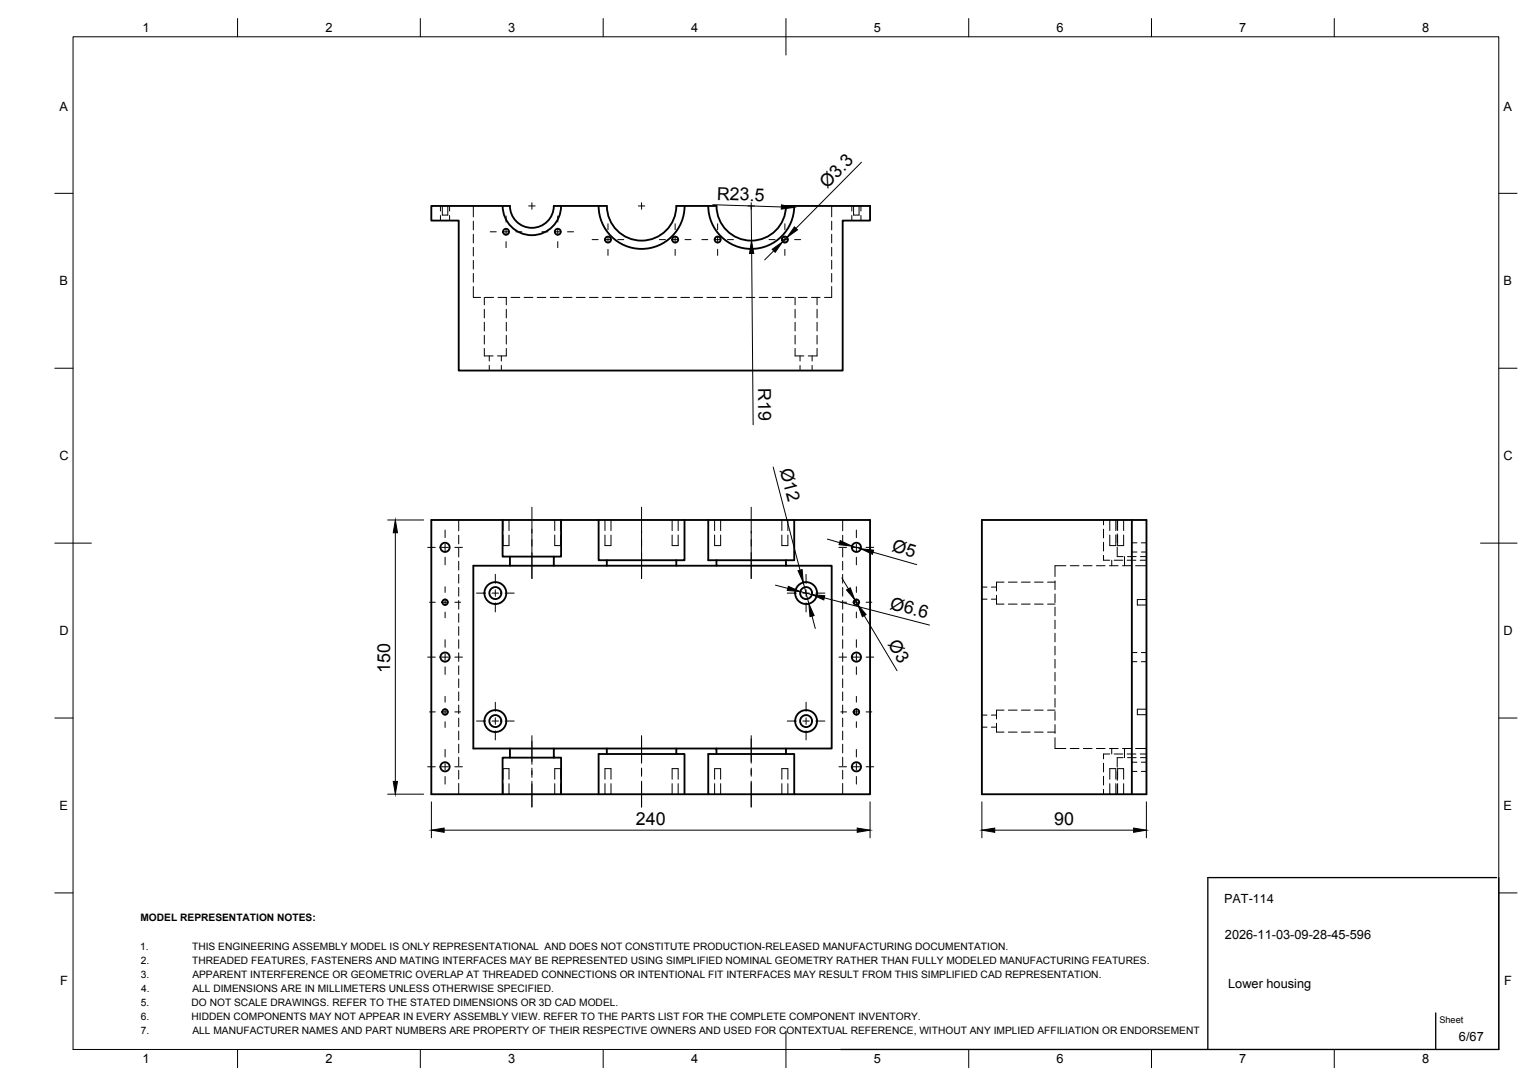
ISO-10303-21;
HEADER;
/* Generated by software containing ST-Developer
 * from STEP Tools, Inc. (www.steptools.com) 
 */

FILE_DESCRIPTION(
/* description */ ('Two-stage gear reducer in split housing'),
/* implementation_level */ '2;1');

FILE_NAME(
/* name */ 'Lower housing.step',
/* time_stamp */ '2026-10-28T03:22:31-07:00',
/* author */ (''),
/* organization */ (''),
/* preprocessor_version */ 'ST-DEVELOPER v20.2',
/* originating_system */ 'Autodesk Translation Framework v15.17.0.0',
/* authorisation */ '');

FILE_SCHEMA (('AUTOMOTIVE_DESIGN { 1 0 10303 214 3 1 1 }'));
ENDSEC;

DATA;
#10=MECHANICAL_DESIGN_GEOMETRIC_PRESENTATION_REPRESENTATION('',(#1235),#73366);
#1123=SHAPE_REPRESENTATION_RELATIONSHIP('SRR','None',#73610,#1179);
#1179=ADVANCED_BREP_SHAPE_REPRESENTATION('',(#1306),#73306);
#1235=STYLED_ITEM('',(#73967),#1306);
#1306=MANIFOLD_SOLID_BREP('Body1',#16123);
#1382=FACE_BOUND('',#2944,.T.);
#1383=FACE_BOUND('',#2945,.T.);
#1384=FACE_BOUND('',#2946,.T.);
#1385=FACE_BOUND('',#2947,.T.);
#1386=FACE_BOUND('',#2948,.T.);
#1387=FACE_BOUND('',#2949,.T.);
#1388=FACE_BOUND('',#2951,.T.);
#1389=FACE_BOUND('',#2952,.T.);
#1390=FACE_BOUND('',#2953,.T.);
#1391=FACE_BOUND('',#2954,.T.);
#1392=FACE_BOUND('',#2955,.T.);
#1393=FACE_BOUND('',#2959,.T.);
#1394=FACE_BOUND('',#2960,.T.);
#1395=FACE_BOUND('',#2961,.T.);
#1396=FACE_BOUND('',#2962,.T.);
#1397=FACE_BOUND('',#2963,.T.);
#1398=FACE_BOUND('',#2964,.T.);
#1399=FACE_BOUND('',#2998,.T.);
#1400=FACE_BOUND('',#2999,.T.);
#1401=FACE_BOUND('',#3000,.T.);
#1402=FACE_BOUND('',#3001,.T.);
#1403=FACE_BOUND('',#3002,.T.);
#1404=FACE_BOUND('',#3009,.T.);
#1405=FACE_BOUND('',#3012,.T.);
#1406=FACE_BOUND('',#3015,.T.);
#1407=FACE_BOUND('',#3018,.T.);
#1408=FACE_BOUND('',#3039,.T.);
#1409=FACE_BOUND('',#3040,.T.);
#1410=FACE_BOUND('',#3041,.T.);
#1411=FACE_BOUND('',#3045,.T.);
#1412=FACE_BOUND('',#3046,.T.);
#1413=FACE_BOUND('',#3047,.T.);
#1414=FACE_BOUND('',#3051,.T.);
#1415=FACE_BOUND('',#3052,.T.);
#1416=FACE_BOUND('',#3053,.T.);
#1417=FACE_BOUND('',#3054,.T.);
#1418=FACE_BOUND('',#3057,.T.);
#1419=FACE_BOUND('',#3058,.T.);
#1420=FACE_BOUND('',#3059,.T.);
#1421=FACE_BOUND('',#3060,.T.);
#1608=PLANE('',#16837);
#1609=PLANE('',#16841);
#1610=PLANE('',#16845);
#1611=PLANE('',#16849);
#1612=PLANE('',#16853);
#1613=PLANE('',#16855);
#1614=PLANE('',#16862);
#1615=PLANE('',#16871);
#1616=PLANE('',#16873);
#1617=PLANE('',#16880);
#1618=PLANE('',#16885);
#1619=PLANE('',#16888);
#1620=PLANE('',#16891);
#1621=PLANE('',#16894);
#1622=PLANE('',#16897);
#1623=PLANE('',#16900);
#1624=PLANE('',#16903);
#1625=PLANE('',#16907);
#1626=PLANE('',#16909);
#1627=PLANE('',#16913);
#1628=PLANE('',#16915);
#1629=PLANE('',#16918);
#1630=PLANE('',#16921);
#1631=PLANE('',#16924);
#1632=PLANE('',#16927);
#1633=PLANE('',#16930);
#1634=PLANE('',#16932);
#1635=PLANE('',#16940);
#1636=PLANE('',#16947);
#1637=PLANE('',#16952);
#1638=PLANE('',#16957);
#1639=PLANE('',#16962);
#1640=PLANE('',#16974);
#1641=PLANE('',#16977);
#1642=PLANE('',#16980);
#1643=PLANE('',#16983);
#1644=PLANE('',#16996);
#1645=PLANE('',#16997);
#1646=PLANE('',#16998);
#1647=PLANE('',#16999);
#1648=PLANE('',#17000);
#1649=PLANE('',#17001);
#1650=PLANE('',#17002);
#1651=PLANE('',#17003);
#1652=PLANE('',#17004);
#1653=PLANE('',#17005);
#2012=FACE_OUTER_BOUND('',#2933,.T.);
#2013=FACE_OUTER_BOUND('',#2934,.T.);
#2014=FACE_OUTER_BOUND('',#2935,.T.);
#2015=FACE_OUTER_BOUND('',#2936,.T.);
#2016=FACE_OUTER_BOUND('',#2937,.T.);
#2017=FACE_OUTER_BOUND('',#2938,.T.);
#2018=FACE_OUTER_BOUND('',#2939,.T.);
#2019=FACE_OUTER_BOUND('',#2940,.T.);
#2020=FACE_OUTER_BOUND('',#2941,.T.);
#2021=FACE_OUTER_BOUND('',#2942,.T.);
#2022=FACE_OUTER_BOUND('',#2943,.T.);
#2023=FACE_OUTER_BOUND('',#2950,.T.);
#2024=FACE_OUTER_BOUND('',#2956,.T.);
#2025=FACE_OUTER_BOUND('',#2957,.T.);
#2026=FACE_OUTER_BOUND('',#2958,.T.);
#2027=FACE_OUTER_BOUND('',#2965,.T.);
#2028=FACE_OUTER_BOUND('',#2966,.T.);
#2029=FACE_OUTER_BOUND('',#2967,.T.);
#2030=FACE_OUTER_BOUND('',#2968,.T.);
#2031=FACE_OUTER_BOUND('',#2969,.T.);
#2032=FACE_OUTER_BOUND('',#2970,.T.);
#2033=FACE_OUTER_BOUND('',#2971,.T.);
#2034=FACE_OUTER_BOUND('',#2972,.T.);
#2035=FACE_OUTER_BOUND('',#2973,.T.);
#2036=FACE_OUTER_BOUND('',#2974,.T.);
#2037=FACE_OUTER_BOUND('',#2975,.T.);
#2038=FACE_OUTER_BOUND('',#2976,.T.);
#2039=FACE_OUTER_BOUND('',#2977,.T.);
#2040=FACE_OUTER_BOUND('',#2978,.T.);
#2041=FACE_OUTER_BOUND('',#2979,.T.);
#2042=FACE_OUTER_BOUND('',#2980,.T.);
#2043=FACE_OUTER_BOUND('',#2981,.T.);
#2044=FACE_OUTER_BOUND('',#2982,.T.);
#2045=FACE_OUTER_BOUND('',#2983,.T.);
#2046=FACE_OUTER_BOUND('',#2984,.T.);
#2047=FACE_OUTER_BOUND('',#2985,.T.);
#2048=FACE_OUTER_BOUND('',#2986,.T.);
#2049=FACE_OUTER_BOUND('',#2987,.T.);
#2050=FACE_OUTER_BOUND('',#2988,.T.);
#2051=FACE_OUTER_BOUND('',#2989,.T.);
#2052=FACE_OUTER_BOUND('',#2990,.T.);
#2053=FACE_OUTER_BOUND('',#2991,.T.);
#2054=FACE_OUTER_BOUND('',#2992,.T.);
#2055=FACE_OUTER_BOUND('',#2993,.T.);
#2056=FACE_OUTER_BOUND('',#2994,.T.);
#2057=FACE_OUTER_BOUND('',#2995,.T.);
#2058=FACE_OUTER_BOUND('',#2996,.T.);
#2059=FACE_OUTER_BOUND('',#2997,.T.);
#2060=FACE_OUTER_BOUND('',#3003,.T.);
#2061=FACE_OUTER_BOUND('',#3004,.T.);
#2062=FACE_OUTER_BOUND('',#3005,.T.);
#2063=FACE_OUTER_BOUND('',#3006,.T.);
#2064=FACE_OUTER_BOUND('',#3007,.T.);
#2065=FACE_OUTER_BOUND('',#3008,.T.);
#2066=FACE_OUTER_BOUND('',#3010,.T.);
#2067=FACE_OUTER_BOUND('',#3011,.T.);
#2068=FACE_OUTER_BOUND('',#3013,.T.);
#2069=FACE_OUTER_BOUND('',#3014,.T.);
#2070=FACE_OUTER_BOUND('',#3016,.T.);
#2071=FACE_OUTER_BOUND('',#3017,.T.);
#2072=FACE_OUTER_BOUND('',#3019,.T.);
#2073=FACE_OUTER_BOUND('',#3020,.T.);
#2074=FACE_OUTER_BOUND('',#3021,.T.);
#2075=FACE_OUTER_BOUND('',#3022,.T.);
#2076=FACE_OUTER_BOUND('',#3023,.T.);
#2077=FACE_OUTER_BOUND('',#3024,.T.);
#2078=FACE_OUTER_BOUND('',#3025,.T.);
#2079=FACE_OUTER_BOUND('',#3026,.T.);
#2080=FACE_OUTER_BOUND('',#3027,.T.);
#2081=FACE_OUTER_BOUND('',#3028,.T.);
#2082=FACE_OUTER_BOUND('',#3029,.T.);
#2083=FACE_OUTER_BOUND('',#3030,.T.);
#2084=FACE_OUTER_BOUND('',#3031,.T.);
#2085=FACE_OUTER_BOUND('',#3032,.T.);
#2086=FACE_OUTER_BOUND('',#3033,.T.);
#2087=FACE_OUTER_BOUND('',#3034,.T.);
#2088=FACE_OUTER_BOUND('',#3035,.T.);
#2089=FACE_OUTER_BOUND('',#3036,.T.);
#2090=FACE_OUTER_BOUND('',#3037,.T.);
#2091=FACE_OUTER_BOUND('',#3038,.T.);
#2092=FACE_OUTER_BOUND('',#3042,.T.);
#2093=FACE_OUTER_BOUND('',#3043,.T.);
#2094=FACE_OUTER_BOUND('',#3044,.T.);
#2095=FACE_OUTER_BOUND('',#3048,.T.);
#2096=FACE_OUTER_BOUND('',#3049,.T.);
#2097=FACE_OUTER_BOUND('',#3050,.T.);
#2098=FACE_OUTER_BOUND('',#3055,.T.);
#2099=FACE_OUTER_BOUND('',#3056,.T.);
#2933=EDGE_LOOP('',(#10555,#10556,#10557,#10558));
#2934=EDGE_LOOP('',(#10559));
#2935=EDGE_LOOP('',(#10560,#10561,#10562,#10563));
#2936=EDGE_LOOP('',(#10564));
#2937=EDGE_LOOP('',(#10565,#10566,#10567,#10568));
#2938=EDGE_LOOP('',(#10569));
#2939=EDGE_LOOP('',(#10570,#10571,#10572,#10573));
#2940=EDGE_LOOP('',(#10574));
#2941=EDGE_LOOP('',(#10575,#10576,#10577,#10578));
#2942=EDGE_LOOP('',(#10579,#10580,#10581,#10582));
#2943=EDGE_LOOP('',(#10583,#10584,#10585,#10586,#10587,#10588,#10589,#10590,
#10591,#10592,#10593,#10594,#10595,#10596));
#2944=EDGE_LOOP('',(#10597));
#2945=EDGE_LOOP('',(#10598));
#2946=EDGE_LOOP('',(#10599));
#2947=EDGE_LOOP('',(#10600));
#2948=EDGE_LOOP('',(#10601));
#2949=EDGE_LOOP('',(#10602));
#2950=EDGE_LOOP('',(#10603,#10604,#10605,#10606,#10607,#10608,#10609,#10610,
#10611,#10612,#10613,#10614));
#2951=EDGE_LOOP('',(#10615));
#2952=EDGE_LOOP('',(#10616));
#2953=EDGE_LOOP('',(#10617));
#2954=EDGE_LOOP('',(#10618));
#2955=EDGE_LOOP('',(#10619));
#2956=EDGE_LOOP('',(#10620,#10621,#10622,#10623));
#2957=EDGE_LOOP('',(#10624,#10625,#10626,#10627));
#2958=EDGE_LOOP('',(#10628,#10629,#10630,#10631,#10632,#10633,#10634,#10635,
#10636,#10637,#10638,#10639,#10640,#10641));
#2959=EDGE_LOOP('',(#10642));
#2960=EDGE_LOOP('',(#10643));
#2961=EDGE_LOOP('',(#10644));
#2962=EDGE_LOOP('',(#10645));
#2963=EDGE_LOOP('',(#10646));
#2964=EDGE_LOOP('',(#10647));
#2965=EDGE_LOOP('',(#10648,#10649,#10650,#10651,#10652,#10653,#10654,#10655));
#2966=EDGE_LOOP('',(#10656,#10657,#10658,#10659));
#2967=EDGE_LOOP('',(#10660,#10661,#10662,#10663));
#2968=EDGE_LOOP('',(#10664,#10665,#10666,#10667,#10668,#10669,#10670,#10671,
#10672,#10673));
#2969=EDGE_LOOP('',(#10674,#10675,#10676,#10677,#10678,#10679,#10680,#10681));
#2970=EDGE_LOOP('',(#10682,#10683,#10684,#10685));
#2971=EDGE_LOOP('',(#10686));
#2972=EDGE_LOOP('',(#10687,#10688,#10689,#10690));
#2973=EDGE_LOOP('',(#10691));
#2974=EDGE_LOOP('',(#10692,#10693,#10694,#10695));
#2975=EDGE_LOOP('',(#10696));
#2976=EDGE_LOOP('',(#10697,#10698,#10699,#10700));
#2977=EDGE_LOOP('',(#10701));
#2978=EDGE_LOOP('',(#10702,#10703,#10704,#10705));
#2979=EDGE_LOOP('',(#10706,#10707,#10708,#10709));
#2980=EDGE_LOOP('',(#10710,#10711,#10712,#10713));
#2981=EDGE_LOOP('',(#10714,#10715,#10716,#10717));
#2982=EDGE_LOOP('',(#10718,#10719,#10720,#10721,#10722,#10723,#10724,#10725));
#2983=EDGE_LOOP('',(#10726,#10727,#10728,#10729));
#2984=EDGE_LOOP('',(#10730,#10731,#10732,#10733));
#2985=EDGE_LOOP('',(#10734,#10735,#10736,#10737,#10738,#10739,#10740,#10741,
#10742,#10743));
#2986=EDGE_LOOP('',(#10744,#10745,#10746,#10747,#10748,#10749,#10750,#10751));
#2987=EDGE_LOOP('',(#10752,#10753,#10754,#10755));
#2988=EDGE_LOOP('',(#10756));
#2989=EDGE_LOOP('',(#10757,#10758,#10759,#10760));
#2990=EDGE_LOOP('',(#10761));
#2991=EDGE_LOOP('',(#10762,#10763,#10764,#10765));
#2992=EDGE_LOOP('',(#10766));
#2993=EDGE_LOOP('',(#10767,#10768,#10769,#10770));
#2994=EDGE_LOOP('',(#10771));
#2995=EDGE_LOOP('',(#10772,#10773,#10774,#10775));
#2996=EDGE_LOOP('',(#10776,#10777,#10778,#10779));
#2997=EDGE_LOOP('',(#10780,#10781,#10782,#10783,#10784,#10785,#10786,#10787,
#10788,#10789,#10790,#10791));
#2998=EDGE_LOOP('',(#10792));
#2999=EDGE_LOOP('',(#10793));
#3000=EDGE_LOOP('',(#10794));
#3001=EDGE_LOOP('',(#10795));
#3002=EDGE_LOOP('',(#10796));
#3003=EDGE_LOOP('',(#10797,#10798,#10799,#10800));
#3004=EDGE_LOOP('',(#10801,#10802,#10803,#10804));
#3005=EDGE_LOOP('',(#10805,#10806,#10807,#10808));
#3006=EDGE_LOOP('',(#10809,#10810,#10811,#10812));
#3007=EDGE_LOOP('',(#10813,#10814,#10815,#10816));
#3008=EDGE_LOOP('',(#10817));
#3009=EDGE_LOOP('',(#10818));
#3010=EDGE_LOOP('',(#10819,#10820,#10821,#10822));
#3011=EDGE_LOOP('',(#10823));
#3012=EDGE_LOOP('',(#10824));
#3013=EDGE_LOOP('',(#10825,#10826,#10827,#10828));
#3014=EDGE_LOOP('',(#10829));
#3015=EDGE_LOOP('',(#10830));
#3016=EDGE_LOOP('',(#10831,#10832,#10833,#10834));
#3017=EDGE_LOOP('',(#10835));
#3018=EDGE_LOOP('',(#10836));
#3019=EDGE_LOOP('',(#10837,#10838,#10839,#10840));
#3020=EDGE_LOOP('',(#10841,#10842,#10843,#10844));
#3021=EDGE_LOOP('',(#10845,#10846,#10847,#10848));
#3022=EDGE_LOOP('',(#10849,#10850,#10851,#10852));
#3023=EDGE_LOOP('',(#10853,#10854,#10855,#10856));
#3024=EDGE_LOOP('',(#10857));
#3025=EDGE_LOOP('',(#10858,#10859,#10860,#10861));
#3026=EDGE_LOOP('',(#10862));
#3027=EDGE_LOOP('',(#10863,#10864,#10865,#10866));
#3028=EDGE_LOOP('',(#10867));
#3029=EDGE_LOOP('',(#10868,#10869,#10870,#10871));
#3030=EDGE_LOOP('',(#10872));
#3031=EDGE_LOOP('',(#10873,#10874,#10875,#10876));
#3032=EDGE_LOOP('',(#10877,#10878,#10879,#10880));
#3033=EDGE_LOOP('',(#10881,#10882,#10883,#10884));
#3034=EDGE_LOOP('',(#10885,#10886,#10887,#10888));
#3035=EDGE_LOOP('',(#10889,#10890,#10891,#10892));
#3036=EDGE_LOOP('',(#10893,#10894,#10895,#10896));
#3037=EDGE_LOOP('',(#10897,#10898,#10899,#10900));
#3038=EDGE_LOOP('',(#10901,#10902,#10903,#10904));
#3039=EDGE_LOOP('',(#10905));
#3040=EDGE_LOOP('',(#10906));
#3041=EDGE_LOOP('',(#10907));
#3042=EDGE_LOOP('',(#10908,#10909,#10910,#10911));
#3043=EDGE_LOOP('',(#10912,#10913,#10914,#10915));
#3044=EDGE_LOOP('',(#10916,#10917,#10918,#10919));
#3045=EDGE_LOOP('',(#10920));
#3046=EDGE_LOOP('',(#10921));
#3047=EDGE_LOOP('',(#10922));
#3048=EDGE_LOOP('',(#10923,#10924,#10925,#10926));
#3049=EDGE_LOOP('',(#10927,#10928,#10929,#10930));
#3050=EDGE_LOOP('',(#10931,#10932,#10933,#10934));
#3051=EDGE_LOOP('',(#10935));
#3052=EDGE_LOOP('',(#10936));
#3053=EDGE_LOOP('',(#10937));
#3054=EDGE_LOOP('',(#10938));
#3055=EDGE_LOOP('',(#10939,#10940,#10941,#10942));
#3056=EDGE_LOOP('',(#10943,#10944,#10945,#10946));
#3057=EDGE_LOOP('',(#10947));
#3058=EDGE_LOOP('',(#10948));
#3059=EDGE_LOOP('',(#10949));
#3060=EDGE_LOOP('',(#10950));
#4072=LINE('',#22832,#5096);
#4073=LINE('',#22839,#5097);
#4074=LINE('',#22846,#5098);
#4075=LINE('',#22853,#5099);
#4076=LINE('',#22859,#5100);
#4077=LINE('',#22863,#5101);
#4078=LINE('',#22867,#5102);
#4079=LINE('',#22870,#5103);
#4080=LINE('',#22873,#5104);
#4081=LINE('',#22875,#5105);
#4082=LINE('',#22877,#5106);
#4083=LINE('',#22879,#5107);
#4084=LINE('',#22881,#5108);
#4085=LINE('',#22883,#5109);
#4086=LINE('',#22885,#5110);
#4087=LINE('',#22887,#5111);
#4088=LINE('',#22889,#5112);
#4089=LINE('',#22893,#5113);
#4090=LINE('',#22896,#5114);
#4091=LINE('',#22907,#5115);
#4092=LINE('',#22909,#5116);
#4093=LINE('',#22911,#5117);
#4094=LINE('',#22913,#5118);
#4095=LINE('',#22915,#5119);
#4096=LINE('',#22917,#5120);
#4097=LINE('',#22919,#5121);
#4098=LINE('',#22921,#5122);
#4099=LINE('',#22922,#5123);
#4100=LINE('',#22937,#5124);
#4101=LINE('',#22942,#5125);
#4102=LINE('',#22945,#5126);
#4103=LINE('',#22949,#5127);
#4104=LINE('',#22953,#5128);
#4105=LINE('',#22955,#5129);
#4106=LINE('',#22957,#5130);
#4107=LINE('',#22959,#5131);
#4108=LINE('',#22961,#5132);
#4109=LINE('',#22963,#5133);
#4110=LINE('',#22965,#5134);
#4111=LINE('',#22966,#5135);
#4112=LINE('',#22977,#5136);
#4113=LINE('',#22979,#5137);
#4114=LINE('',#22981,#5138);
#4115=LINE('',#22983,#5139);
#4116=LINE('',#22984,#5140);
#4117=LINE('',#22989,#5141);
#4118=LINE('',#22993,#5142);
#4119=LINE('',#22997,#5143);
#4120=LINE('',#23001,#5144);
#4121=LINE('',#23003,#5145);
#4122=LINE('',#23005,#5146);
#4123=LINE('',#23006,#5147);
#4124=LINE('',#23009,#5148);
#4125=LINE('',#23011,#5149);
#4126=LINE('',#23012,#5150);
#4127=LINE('',#23016,#5151);
#4128=LINE('',#23021,#5152);
#4129=LINE('',#23025,#5153);
#4130=LINE('',#23030,#5154);
#4131=LINE('',#23035,#5155);
#4132=LINE('',#23039,#5156);
#4133=LINE('',#23044,#5157);
#4134=LINE('',#23048,#5158);
#4135=LINE('',#23051,#5159);
#4136=LINE('',#23053,#5160);
#4137=LINE('',#23055,#5161);
#4138=LINE('',#23057,#5162);
#4139=LINE('',#23058,#5163);
#4140=LINE('',#23060,#5164);
#4141=LINE('',#23065,#5165);
#4142=LINE('',#23067,#5166);
#4143=LINE('',#23069,#5167);
#4144=LINE('',#23071,#5168);
#4145=LINE('',#23075,#5169);
#4146=LINE('',#23077,#5170);
#4147=LINE('',#23078,#5171);
#4148=LINE('',#23082,#5172);
#4149=LINE('',#23087,#5173);
#4150=LINE('',#23091,#5174);
#4151=LINE('',#23096,#5175);
#4152=LINE('',#23101,#5176);
#4153=LINE('',#23105,#5177);
#4154=LINE('',#23108,#5178);
#4155=LINE('',#23110,#5179);
#4156=LINE('',#23112,#5180);
#4157=LINE('',#23113,#5181);
#4158=LINE('',#23114,#5182);
#4159=LINE('',#23115,#5183);
#4160=LINE('',#23136,#5184);
#4161=LINE('',#23145,#5185);
#4162=LINE('',#23154,#5186);
#4163=LINE('',#23163,#5187);
#4164=LINE('',#23171,#5188);
#4165=LINE('',#23175,#5189);
#4166=LINE('',#23179,#5190);
#4167=LINE('',#23183,#5191);
#4168=LINE('',#23187,#5192);
#4169=LINE('',#23192,#5193);
#4170=LINE('',#23197,#5194);
#4171=LINE('',#23202,#5195);
#4172=LINE('',#23207,#5196);
#4173=LINE('',#23211,#5197);
#4174=LINE('',#23215,#5198);
#4175=LINE('',#23219,#5199);
#4176=LINE('',#23223,#5200);
#4177=LINE('',#23227,#5201);
#4178=LINE('',#23229,#5202);
#4179=LINE('',#23231,#5203);
#4180=LINE('',#23233,#5204);
#4181=LINE('',#23235,#5205);
#4182=LINE('',#23237,#5206);
#4183=LINE('',#23239,#5207);
#4184=LINE('',#23241,#5208);
#4185=LINE('',#23244,#5209);
#5096=VECTOR('',#18522,0.164999999999999);
#5097=VECTOR('',#18531,0.164999999999999);
#5098=VECTOR('',#18540,0.164999999999999);
#5099=VECTOR('',#18549,0.164999999999999);
#5100=VECTOR('',#18556,1.);
#5101=VECTOR('',#18559,1.);
#5102=VECTOR('',#18564,1.);
#5103=VECTOR('',#18567,1.);
#5104=VECTOR('',#18570,1.);
#5105=VECTOR('',#18571,1.);
#5106=VECTOR('',#18572,1.);
#5107=VECTOR('',#18573,1.);
#5108=VECTOR('',#18574,1.);
#5109=VECTOR('',#18575,1.);
#5110=VECTOR('',#18576,1.);
#5111=VECTOR('',#18577,1.);
#5112=VECTOR('',#18578,1.);
#5113=VECTOR('',#18581,1.);
#5114=VECTOR('',#18584,1.);
#5115=VECTOR('',#18595,1.);
#5116=VECTOR('',#18596,1.);
#5117=VECTOR('',#18597,1.);
#5118=VECTOR('',#18598,1.);
#5119=VECTOR('',#18599,1.);
#5120=VECTOR('',#18600,1.);
#5121=VECTOR('',#18601,1.);
#5122=VECTOR('',#18602,1.);
#5123=VECTOR('',#18603,1.);
#5124=VECTOR('',#18618,1.);
#5125=VECTOR('',#18625,1.);
#5126=VECTOR('',#18628,1.);
#5127=VECTOR('',#18631,1.);
#5128=VECTOR('',#18634,1.);
#5129=VECTOR('',#18635,1.);
#5130=VECTOR('',#18636,1.);
#5131=VECTOR('',#18637,1.);
#5132=VECTOR('',#18638,1.);
#5133=VECTOR('',#18639,1.);
#5134=VECTOR('',#18640,1.);
#5135=VECTOR('',#18641,1.);
#5136=VECTOR('',#18652,1.);
#5137=VECTOR('',#18653,1.);
#5138=VECTOR('',#18654,1.);
#5139=VECTOR('',#18655,1.);
#5140=VECTOR('',#18656,1.);
#5141=VECTOR('',#18663,1.);
#5142=VECTOR('',#18668,1.);
#5143=VECTOR('',#18671,1.);
#5144=VECTOR('',#18674,1.);
#5145=VECTOR('',#18675,1.);
#5146=VECTOR('',#18676,1.);
#5147=VECTOR('',#18677,1.);
#5148=VECTOR('',#18680,1.);
#5149=VECTOR('',#18681,1.);
#5150=VECTOR('',#18682,1.);
#5151=VECTOR('',#18687,0.165);
#5152=VECTOR('',#18694,0.165);
#5153=VECTOR('',#18699,0.165);
#5154=VECTOR('',#18706,0.165);
#5155=VECTOR('',#18713,1.);
#5156=VECTOR('',#18718,1.);
#5157=VECTOR('',#18725,1.);
#5158=VECTOR('',#18730,1.);
#5159=VECTOR('',#18733,1.);
#5160=VECTOR('',#18734,1.);
#5161=VECTOR('',#18735,1.);
#5162=VECTOR('',#18736,1.);
#5163=VECTOR('',#18737,1.);
#5164=VECTOR('',#18740,1.);
#5165=VECTOR('',#18747,1.);
#5166=VECTOR('',#18748,1.);
#5167=VECTOR('',#18749,1.);
#5168=VECTOR('',#18750,1.);
#5169=VECTOR('',#18755,1.);
#5170=VECTOR('',#18756,1.);
#5171=VECTOR('',#18757,1.);
#5172=VECTOR('',#18762,0.165);
#5173=VECTOR('',#18769,0.165);
#5174=VECTOR('',#18774,0.165);
#5175=VECTOR('',#18781,0.165);
#5176=VECTOR('',#18788,1.);
#5177=VECTOR('',#18793,1.);
#5178=VECTOR('',#18798,1.);
#5179=VECTOR('',#18799,1.);
#5180=VECTOR('',#18800,1.);
#5181=VECTOR('',#18801,1.);
#5182=VECTOR('',#18802,1.);
#5183=VECTOR('',#18803,1.);
#5184=VECTOR('',#18830,0.6);
#5185=VECTOR('',#18841,0.6);
#5186=VECTOR('',#18852,0.6);
#5187=VECTOR('',#18863,0.6);
#5188=VECTOR('',#18874,0.33);
#5189=VECTOR('',#18879,0.33);
#5190=VECTOR('',#18884,0.33);
#5191=VECTOR('',#18889,0.33);
#5192=VECTOR('',#18894,0.149999999999999);
#5193=VECTOR('',#18901,0.149999999999999);
#5194=VECTOR('',#18908,0.15);
#5195=VECTOR('',#18915,0.15);
#5196=VECTOR('',#18922,0.25);
#5197=VECTOR('',#18927,0.25);
#5198=VECTOR('',#18932,0.25);
#5199=VECTOR('',#18937,0.25);
#5200=VECTOR('',#18942,0.25);
#5201=VECTOR('',#18947,0.25);
#5202=VECTOR('',#18950,1.);
#5203=VECTOR('',#18953,1.);
#5204=VECTOR('',#18956,1.);
#5205=VECTOR('',#18959,1.);
#5206=VECTOR('',#18962,1.);
#5207=VECTOR('',#18965,1.);
#5208=VECTOR('',#18968,1.);
#5209=VECTOR('',#18973,1.);
#6112=CIRCLE('',#16835,0.164999999999999);
#6113=CIRCLE('',#16836,0.164999999999999);
#6114=CIRCLE('',#16839,0.164999999999999);
#6115=CIRCLE('',#16840,0.164999999999999);
#6116=CIRCLE('',#16843,0.164999999999999);
#6117=CIRCLE('',#16844,0.164999999999999);
#6118=CIRCLE('',#16847,0.164999999999999);
#6119=CIRCLE('',#16848,0.164999999999999);
#6120=CIRCLE('',#16851,2.35);
#6121=CIRCLE('',#16852,2.35);
#6122=CIRCLE('',#16854,1.9);
#6123=CIRCLE('',#16856,1.6);
#6124=CIRCLE('',#16857,2.35);
#6125=CIRCLE('',#16858,0.165);
#6126=CIRCLE('',#16859,0.165);
#6127=CIRCLE('',#16860,0.165);
#6128=CIRCLE('',#16861,0.165);
#6129=CIRCLE('',#16863,0.149999999999999);
#6130=CIRCLE('',#16864,0.25);
#6131=CIRCLE('',#16865,0.25);
#6132=CIRCLE('',#16866,0.25);
#6133=CIRCLE('',#16867,0.149999999999999);
#6134=CIRCLE('',#16869,2.35);
#6135=CIRCLE('',#16870,2.35);
#6136=CIRCLE('',#16872,1.9);
#6137=CIRCLE('',#16874,2.35);
#6138=CIRCLE('',#16875,1.6);
#6139=CIRCLE('',#16876,0.165);
#6140=CIRCLE('',#16877,0.165);
#6141=CIRCLE('',#16878,0.165);
#6142=CIRCLE('',#16879,0.165);
#6143=CIRCLE('',#16882,1.9);
#6144=CIRCLE('',#16884,1.9);
#6145=CIRCLE('',#16886,1.9);
#6146=CIRCLE('',#16887,1.2);
#6147=CIRCLE('',#16890,0.165);
#6148=CIRCLE('',#16893,0.165);
#6149=CIRCLE('',#16896,0.165);
#6150=CIRCLE('',#16899,0.165);
#6151=CIRCLE('',#16902,2.35);
#6152=CIRCLE('',#16904,1.9);
#6153=CIRCLE('',#16906,2.35);
#6154=CIRCLE('',#16908,1.9);
#6155=CIRCLE('',#16912,1.9);
#6156=CIRCLE('',#16914,1.2);
#6157=CIRCLE('',#16917,0.165);
#6158=CIRCLE('',#16920,0.165);
#6159=CIRCLE('',#16923,0.165);
#6160=CIRCLE('',#16926,0.165);
#6161=CIRCLE('',#16929,1.6);
#6162=CIRCLE('',#16931,1.2);
#6163=CIRCLE('',#16933,0.15);
#6164=CIRCLE('',#16934,0.25);
#6165=CIRCLE('',#16935,0.25);
#6166=CIRCLE('',#16936,0.25);
#6167=CIRCLE('',#16937,0.15);
#6168=CIRCLE('',#16939,1.6);
#6169=CIRCLE('',#16941,1.2);
#6170=CIRCLE('',#16945,0.6);
#6171=CIRCLE('',#16946,0.6);
#6172=CIRCLE('',#16948,0.33);
#6173=CIRCLE('',#16950,0.6);
#6174=CIRCLE('',#16951,0.6);
#6175=CIRCLE('',#16953,0.33);
#6176=CIRCLE('',#16955,0.6);
#6177=CIRCLE('',#16956,0.6);
#6178=CIRCLE('',#16958,0.33);
#6179=CIRCLE('',#16960,0.6);
#6180=CIRCLE('',#16961,0.6);
#6181=CIRCLE('',#16963,0.33);
#6182=CIRCLE('',#16965,0.33);
#6183=CIRCLE('',#16967,0.33);
#6184=CIRCLE('',#16969,0.33);
#6185=CIRCLE('',#16971,0.33);
#6186=CIRCLE('',#16973,0.149999999999999);
#6187=CIRCLE('',#16976,0.149999999999999);
#6188=CIRCLE('',#16979,0.15);
#6189=CIRCLE('',#16982,0.15);
#6190=CIRCLE('',#16985,0.25);
#6191=CIRCLE('',#16987,0.25);
#6192=CIRCLE('',#16989,0.25);
#6193=CIRCLE('',#16991,0.25);
#6194=CIRCLE('',#16993,0.25);
#6195=CIRCLE('',#16995,0.25);
#6840=VERTEX_POINT('',#22829);
#6841=VERTEX_POINT('',#22831);
#6842=VERTEX_POINT('',#22836);
#6843=VERTEX_POINT('',#22838);
#6844=VERTEX_POINT('',#22843);
#6845=VERTEX_POINT('',#22845);
#6846=VERTEX_POINT('',#22850);
#6847=VERTEX_POINT('',#22852);
#6848=VERTEX_POINT('',#22857);
#6849=VERTEX_POINT('',#22858);
#6850=VERTEX_POINT('',#22860);
#6851=VERTEX_POINT('',#22862);
#6852=VERTEX_POINT('',#22866);
#6853=VERTEX_POINT('',#22868);
#6854=VERTEX_POINT('',#22872);
#6855=VERTEX_POINT('',#22874);
#6856=VERTEX_POINT('',#22876);
#6857=VERTEX_POINT('',#22878);
#6858=VERTEX_POINT('',#22880);
#6859=VERTEX_POINT('',#22882);
#6860=VERTEX_POINT('',#22884);
#6861=VERTEX_POINT('',#22886);
#6862=VERTEX_POINT('',#22888);
#6863=VERTEX_POINT('',#22890);
#6864=VERTEX_POINT('',#22892);
#6865=VERTEX_POINT('',#22894);
#6866=VERTEX_POINT('',#22897);
#6867=VERTEX_POINT('',#22899);
#6868=VERTEX_POINT('',#22901);
#6869=VERTEX_POINT('',#22903);
#6870=VERTEX_POINT('',#22906);
#6871=VERTEX_POINT('',#22908);
#6872=VERTEX_POINT('',#22910);
#6873=VERTEX_POINT('',#22912);
#6874=VERTEX_POINT('',#22914);
#6875=VERTEX_POINT('',#22916);
#6876=VERTEX_POINT('',#22918);
#6877=VERTEX_POINT('',#22920);
#6878=VERTEX_POINT('',#22923);
#6879=VERTEX_POINT('',#22925);
#6880=VERTEX_POINT('',#22927);
#6881=VERTEX_POINT('',#22929);
#6882=VERTEX_POINT('',#22931);
#6883=VERTEX_POINT('',#22934);
#6884=VERTEX_POINT('',#22936);
#6885=VERTEX_POINT('',#22940);
#6886=VERTEX_POINT('',#22944);
#6887=VERTEX_POINT('',#22946);
#6888=VERTEX_POINT('',#22948);
#6889=VERTEX_POINT('',#22950);
#6890=VERTEX_POINT('',#22952);
#6891=VERTEX_POINT('',#22954);
#6892=VERTEX_POINT('',#22956);
#6893=VERTEX_POINT('',#22958);
#6894=VERTEX_POINT('',#22960);
#6895=VERTEX_POINT('',#22962);
#6896=VERTEX_POINT('',#22964);
#6897=VERTEX_POINT('',#22967);
#6898=VERTEX_POINT('',#22969);
#6899=VERTEX_POINT('',#22971);
#6900=VERTEX_POINT('',#22973);
#6901=VERTEX_POINT('',#22976);
#6902=VERTEX_POINT('',#22978);
#6903=VERTEX_POINT('',#22980);
#6904=VERTEX_POINT('',#22982);
#6905=VERTEX_POINT('',#22988);
#6906=VERTEX_POINT('',#22992);
#6907=VERTEX_POINT('',#22994);
#6908=VERTEX_POINT('',#22996);
#6909=VERTEX_POINT('',#22998);
#6910=VERTEX_POINT('',#23000);
#6911=VERTEX_POINT('',#23002);
#6912=VERTEX_POINT('',#23004);
#6913=VERTEX_POINT('',#23008);
#6914=VERTEX_POINT('',#23010);
#6915=VERTEX_POINT('',#23014);
#6916=VERTEX_POINT('',#23019);
#6917=VERTEX_POINT('',#23024);
#6918=VERTEX_POINT('',#23029);
#6919=VERTEX_POINT('',#23034);
#6920=VERTEX_POINT('',#23038);
#6921=VERTEX_POINT('',#23042);
#6922=VERTEX_POINT('',#23046);
#6923=VERTEX_POINT('',#23050);
#6924=VERTEX_POINT('',#23052);
#6925=VERTEX_POINT('',#23054);
#6926=VERTEX_POINT('',#23056);
#6927=VERTEX_POINT('',#23064);
#6928=VERTEX_POINT('',#23066);
#6929=VERTEX_POINT('',#23068);
#6930=VERTEX_POINT('',#23070);
#6931=VERTEX_POINT('',#23074);
#6932=VERTEX_POINT('',#23076);
#6933=VERTEX_POINT('',#23080);
#6934=VERTEX_POINT('',#23085);
#6935=VERTEX_POINT('',#23090);
#6936=VERTEX_POINT('',#23095);
#6937=VERTEX_POINT('',#23100);
#6938=VERTEX_POINT('',#23104);
#6939=VERTEX_POINT('',#23109);
#6940=VERTEX_POINT('',#23111);
#6941=VERTEX_POINT('',#23116);
#6942=VERTEX_POINT('',#23118);
#6943=VERTEX_POINT('',#23120);
#6944=VERTEX_POINT('',#23122);
#6945=VERTEX_POINT('',#23124);
#6946=VERTEX_POINT('',#23133);
#6947=VERTEX_POINT('',#23135);
#6948=VERTEX_POINT('',#23139);
#6949=VERTEX_POINT('',#23142);
#6950=VERTEX_POINT('',#23144);
#6951=VERTEX_POINT('',#23148);
#6952=VERTEX_POINT('',#23151);
#6953=VERTEX_POINT('',#23153);
#6954=VERTEX_POINT('',#23157);
#6955=VERTEX_POINT('',#23160);
#6956=VERTEX_POINT('',#23162);
#6957=VERTEX_POINT('',#23166);
#6958=VERTEX_POINT('',#23169);
#6959=VERTEX_POINT('',#23173);
#6960=VERTEX_POINT('',#23177);
#6961=VERTEX_POINT('',#23181);
#6962=VERTEX_POINT('',#23185);
#6963=VERTEX_POINT('',#23190);
#6964=VERTEX_POINT('',#23195);
#6965=VERTEX_POINT('',#23200);
#6966=VERTEX_POINT('',#23205);
#6967=VERTEX_POINT('',#23209);
#6968=VERTEX_POINT('',#23213);
#6969=VERTEX_POINT('',#23217);
#6970=VERTEX_POINT('',#23221);
#6971=VERTEX_POINT('',#23225);
#8331=EDGE_CURVE('',#6840,#6840,#6112,.T.);
#8332=EDGE_CURVE('',#6840,#6841,#4072,.T.);
#8333=EDGE_CURVE('',#6841,#6841,#6113,.T.);
#8334=EDGE_CURVE('',#6842,#6842,#6114,.T.);
#8335=EDGE_CURVE('',#6842,#6843,#4073,.T.);
#8336=EDGE_CURVE('',#6843,#6843,#6115,.T.);
#8337=EDGE_CURVE('',#6844,#6844,#6116,.T.);
#8338=EDGE_CURVE('',#6844,#6845,#4074,.T.);
#8339=EDGE_CURVE('',#6845,#6845,#6117,.T.);
#8340=EDGE_CURVE('',#6846,#6846,#6118,.T.);
#8341=EDGE_CURVE('',#6846,#6847,#4075,.T.);
#8342=EDGE_CURVE('',#6847,#6847,#6119,.T.);
#8343=EDGE_CURVE('',#6848,#6849,#4076,.T.);
#8344=EDGE_CURVE('',#6850,#6848,#6120,.T.);
#8345=EDGE_CURVE('',#6851,#6850,#4077,.T.);
#8346=EDGE_CURVE('',#6849,#6851,#6121,.T.);
#8347=EDGE_CURVE('',#6852,#6848,#4078,.T.);
#8348=EDGE_CURVE('',#6853,#6852,#6122,.T.);
#8349=EDGE_CURVE('',#6850,#6853,#4079,.T.);
#8350=EDGE_CURVE('',#6854,#6851,#4080,.T.);
#8351=EDGE_CURVE('',#6855,#6854,#4081,.T.);
#8352=EDGE_CURVE('',#6855,#6856,#4082,.T.);
#8353=EDGE_CURVE('',#6857,#6856,#4083,.T.);
#8354=EDGE_CURVE('',#6857,#6858,#4084,.T.);
#8355=EDGE_CURVE('',#6858,#6859,#4085,.T.);
#8356=EDGE_CURVE('',#6859,#6860,#4086,.T.);
#8357=EDGE_CURVE('',#6860,#6861,#4087,.T.);
#8358=EDGE_CURVE('',#6862,#6861,#4088,.T.);
#8359=EDGE_CURVE('',#6862,#6863,#6123,.T.);
#8360=EDGE_CURVE('',#6864,#6863,#4089,.T.);
#8361=EDGE_CURVE('',#6864,#6865,#6124,.T.);
#8362=EDGE_CURVE('',#6849,#6865,#4090,.T.);
#8363=EDGE_CURVE('',#6866,#6866,#6125,.T.);
#8364=EDGE_CURVE('',#6867,#6867,#6126,.T.);
#8365=EDGE_CURVE('',#6868,#6868,#6127,.T.);
#8366=EDGE_CURVE('',#6869,#6869,#6128,.T.);
#8367=EDGE_CURVE('',#6853,#6870,#4091,.T.);
#8368=EDGE_CURVE('',#6870,#6871,#4092,.T.);
#8369=EDGE_CURVE('',#6871,#6872,#4093,.T.);
#8370=EDGE_CURVE('',#6872,#6873,#4094,.T.);
#8371=EDGE_CURVE('',#6873,#6874,#4095,.T.);
#8372=EDGE_CURVE('',#6874,#6875,#4096,.T.);
#8373=EDGE_CURVE('',#6875,#6876,#4097,.T.);
#8374=EDGE_CURVE('',#6876,#6877,#4098,.T.);
#8375=EDGE_CURVE('',#6877,#6854,#4099,.T.);
#8376=EDGE_CURVE('',#6878,#6878,#6129,.T.);
#8377=EDGE_CURVE('',#6879,#6879,#6130,.T.);
#8378=EDGE_CURVE('',#6880,#6880,#6131,.T.);
#8379=EDGE_CURVE('',#6881,#6881,#6132,.T.);
#8380=EDGE_CURVE('',#6882,#6882,#6133,.T.);
#8381=EDGE_CURVE('',#6875,#6883,#6134,.T.);
#8382=EDGE_CURVE('',#6884,#6883,#4100,.T.);
#8383=EDGE_CURVE('',#6876,#6884,#6135,.T.);
#8384=EDGE_CURVE('',#6885,#6874,#6136,.T.);
#8385=EDGE_CURVE('',#6883,#6885,#4101,.T.);
#8386=EDGE_CURVE('',#6886,#6884,#4102,.T.);
#8387=EDGE_CURVE('',#6886,#6887,#6137,.T.);
#8388=EDGE_CURVE('',#6888,#6887,#4103,.T.);
#8389=EDGE_CURVE('',#6888,#6889,#6138,.T.);
#8390=EDGE_CURVE('',#6890,#6889,#4104,.T.);
#8391=EDGE_CURVE('',#6891,#6890,#4105,.T.);
#8392=EDGE_CURVE('',#6891,#6892,#4106,.T.);
#8393=EDGE_CURVE('',#6893,#6892,#4107,.T.);
#8394=EDGE_CURVE('',#6893,#6894,#4108,.T.);
#8395=EDGE_CURVE('',#6894,#6895,#4109,.T.);
#8396=EDGE_CURVE('',#6895,#6896,#4110,.T.);
#8397=EDGE_CURVE('',#6896,#6877,#4111,.T.);
#8398=EDGE_CURVE('',#6897,#6897,#6139,.T.);
#8399=EDGE_CURVE('',#6898,#6898,#6140,.T.);
#8400=EDGE_CURVE('',#6899,#6899,#6141,.T.);
#8401=EDGE_CURVE('',#6900,#6900,#6142,.T.);
#8402=EDGE_CURVE('',#6885,#6901,#4112,.T.);
#8403=EDGE_CURVE('',#6901,#6902,#4113,.T.);
#8404=EDGE_CURVE('',#6902,#6903,#4114,.T.);
#8405=EDGE_CURVE('',#6903,#6904,#4115,.T.);
#8406=EDGE_CURVE('',#6904,#6886,#4116,.T.);
#8407=EDGE_CURVE('',#6901,#6873,#6143,.T.);
#8408=EDGE_CURVE('',#6905,#6852,#4117,.T.);
#8409=EDGE_CURVE('',#6870,#6905,#6144,.T.);
#8410=EDGE_CURVE('',#6906,#6905,#4118,.T.);
#8411=EDGE_CURVE('',#6906,#6907,#6145,.T.);
#8412=EDGE_CURVE('',#6908,#6907,#4119,.T.);
#8413=EDGE_CURVE('',#6908,#6909,#6146,.T.);
#8414=EDGE_CURVE('',#6910,#6909,#4120,.T.);
#8415=EDGE_CURVE('',#6911,#6910,#4121,.T.);
#8416=EDGE_CURVE('',#6912,#6911,#4122,.T.);
#8417=EDGE_CURVE('',#6912,#6871,#4123,.T.);
#8418=EDGE_CURVE('',#6865,#6913,#4124,.T.);
#8419=EDGE_CURVE('',#6913,#6914,#4125,.T.);
#8420=EDGE_CURVE('',#6914,#6906,#4126,.T.);
#8421=EDGE_CURVE('',#6915,#6915,#6147,.T.);
#8422=EDGE_CURVE('',#6915,#6869,#4127,.T.);
#8423=EDGE_CURVE('',#6916,#6916,#6148,.T.);
#8424=EDGE_CURVE('',#6916,#6868,#4128,.T.);
#8425=EDGE_CURVE('',#6897,#6917,#4129,.T.);
#8426=EDGE_CURVE('',#6917,#6917,#6149,.T.);
#8427=EDGE_CURVE('',#6898,#6918,#4130,.T.);
#8428=EDGE_CURVE('',#6918,#6918,#6150,.T.);
#8429=EDGE_CURVE('',#6919,#6864,#4131,.T.);
#8430=EDGE_CURVE('',#6913,#6919,#6151,.T.);
#8431=EDGE_CURVE('',#6920,#6919,#4132,.T.);
#8432=EDGE_CURVE('',#6914,#6920,#6152,.T.);
#8433=EDGE_CURVE('',#6904,#6921,#6153,.T.);
#8434=EDGE_CURVE('',#6887,#6921,#4133,.T.);
#8435=EDGE_CURVE('',#6922,#6903,#6154,.T.);
#8436=EDGE_CURVE('',#6921,#6922,#4134,.T.);
#8437=EDGE_CURVE('',#6922,#6923,#4135,.T.);
#8438=EDGE_CURVE('',#6923,#6924,#4136,.T.);
#8439=EDGE_CURVE('',#6924,#6925,#4137,.T.);
#8440=EDGE_CURVE('',#6925,#6926,#4138,.T.);
#8441=EDGE_CURVE('',#6926,#6888,#4139,.T.);
#8442=EDGE_CURVE('',#6907,#6920,#4140,.T.);
#8443=EDGE_CURVE('',#6923,#6902,#6155,.T.);
#8444=EDGE_CURVE('',#6927,#6872,#4141,.T.);
#8445=EDGE_CURVE('',#6928,#6927,#4142,.T.);
#8446=EDGE_CURVE('',#6928,#6929,#4143,.T.);
#8447=EDGE_CURVE('',#6930,#6929,#4144,.T.);
#8448=EDGE_CURVE('',#6930,#6924,#6156,.T.);
#8449=EDGE_CURVE('',#6863,#6931,#4145,.T.);
#8450=EDGE_CURVE('',#6931,#6932,#4146,.T.);
#8451=EDGE_CURVE('',#6932,#6908,#4147,.T.);
#8452=EDGE_CURVE('',#6933,#6933,#6157,.T.);
#8453=EDGE_CURVE('',#6933,#6867,#4148,.T.);
#8454=EDGE_CURVE('',#6934,#6934,#6158,.T.);
#8455=EDGE_CURVE('',#6934,#6866,#4149,.T.);
#8456=EDGE_CURVE('',#6900,#6935,#4150,.T.);
#8457=EDGE_CURVE('',#6935,#6935,#6159,.T.);
#8458=EDGE_CURVE('',#6899,#6936,#4151,.T.);
#8459=EDGE_CURVE('',#6936,#6936,#6160,.T.);
#8460=EDGE_CURVE('',#6937,#6862,#4152,.T.);
#8461=EDGE_CURVE('',#6931,#6937,#6161,.T.);
#8462=EDGE_CURVE('',#6938,#6937,#4153,.T.);
#8463=EDGE_CURVE('',#6932,#6938,#6162,.T.);
#8464=EDGE_CURVE('',#6861,#6890,#4154,.T.);
#8465=EDGE_CURVE('',#6889,#6939,#4155,.T.);
#8466=EDGE_CURVE('',#6939,#6940,#4156,.T.);
#8467=EDGE_CURVE('',#6940,#6930,#4157,.T.);
#8468=EDGE_CURVE('',#6929,#6910,#4158,.T.);
#8469=EDGE_CURVE('',#6909,#6938,#4159,.T.);
#8470=EDGE_CURVE('',#6941,#6941,#6163,.T.);
#8471=EDGE_CURVE('',#6942,#6942,#6164,.T.);
#8472=EDGE_CURVE('',#6943,#6943,#6165,.T.);
#8473=EDGE_CURVE('',#6944,#6944,#6166,.T.);
#8474=EDGE_CURVE('',#6945,#6945,#6167,.T.);
#8475=EDGE_CURVE('',#6926,#6939,#6168,.T.);
#8476=EDGE_CURVE('',#6940,#6925,#6169,.T.);
#8477=EDGE_CURVE('',#6946,#6946,#6170,.T.);
#8478=EDGE_CURVE('',#6946,#6947,#4160,.T.);
#8479=EDGE_CURVE('',#6947,#6947,#6171,.T.);
#8480=EDGE_CURVE('',#6948,#6948,#6172,.T.);
#8481=EDGE_CURVE('',#6949,#6949,#6173,.T.);
#8482=EDGE_CURVE('',#6949,#6950,#4161,.T.);
#8483=EDGE_CURVE('',#6950,#6950,#6174,.T.);
#8484=EDGE_CURVE('',#6951,#6951,#6175,.T.);
#8485=EDGE_CURVE('',#6952,#6952,#6176,.T.);
#8486=EDGE_CURVE('',#6952,#6953,#4162,.T.);
#8487=EDGE_CURVE('',#6953,#6953,#6177,.T.);
#8488=EDGE_CURVE('',#6954,#6954,#6178,.T.);
#8489=EDGE_CURVE('',#6955,#6955,#6179,.T.);
#8490=EDGE_CURVE('',#6955,#6956,#4163,.T.);
#8491=EDGE_CURVE('',#6956,#6956,#6180,.T.);
#8492=EDGE_CURVE('',#6957,#6957,#6181,.T.);
#8493=EDGE_CURVE('',#6958,#6958,#6182,.T.);
#8494=EDGE_CURVE('',#6958,#6948,#4164,.T.);
#8495=EDGE_CURVE('',#6959,#6959,#6183,.T.);
#8496=EDGE_CURVE('',#6959,#6951,#4165,.T.);
#8497=EDGE_CURVE('',#6960,#6960,#6184,.T.);
#8498=EDGE_CURVE('',#6960,#6954,#4166,.T.);
#8499=EDGE_CURVE('',#6961,#6961,#6185,.T.);
#8500=EDGE_CURVE('',#6961,#6957,#4167,.T.);
#8501=EDGE_CURVE('',#6962,#6962,#6186,.T.);
#8502=EDGE_CURVE('',#6962,#6878,#4168,.T.);
#8503=EDGE_CURVE('',#6963,#6963,#6187,.T.);
#8504=EDGE_CURVE('',#6963,#6882,#4169,.T.);
#8505=EDGE_CURVE('',#6964,#6964,#6188,.T.);
#8506=EDGE_CURVE('',#6964,#6941,#4170,.T.);
#8507=EDGE_CURVE('',#6965,#6965,#6189,.T.);
#8508=EDGE_CURVE('',#6965,#6945,#4171,.T.);
#8509=EDGE_CURVE('',#6966,#6966,#6190,.T.);
#8510=EDGE_CURVE('',#6966,#6879,#4172,.T.);
#8511=EDGE_CURVE('',#6967,#6967,#6191,.T.);
#8512=EDGE_CURVE('',#6967,#6942,#4173,.T.);
#8513=EDGE_CURVE('',#6968,#6968,#6192,.T.);
#8514=EDGE_CURVE('',#6968,#6943,#4174,.T.);
#8515=EDGE_CURVE('',#6969,#6969,#6193,.T.);
#8516=EDGE_CURVE('',#6969,#6944,#4175,.T.);
#8517=EDGE_CURVE('',#6970,#6970,#6194,.T.);
#8518=EDGE_CURVE('',#6970,#6880,#4176,.T.);
#8519=EDGE_CURVE('',#6971,#6971,#6195,.T.);
#8520=EDGE_CURVE('',#6971,#6881,#4177,.T.);
#8521=EDGE_CURVE('',#6896,#6855,#4178,.T.);
#8522=EDGE_CURVE('',#6856,#6895,#4179,.T.);
#8523=EDGE_CURVE('',#6894,#6857,#4180,.T.);
#8524=EDGE_CURVE('',#6860,#6891,#4181,.T.);
#8525=EDGE_CURVE('',#6892,#6859,#4182,.T.);
#8526=EDGE_CURVE('',#6911,#6928,#4183,.T.);
#8527=EDGE_CURVE('',#6927,#6912,#4184,.T.);
#8528=EDGE_CURVE('',#6858,#6893,#4185,.T.);
#10555=ORIENTED_EDGE('',*,*,#8331,.F.);
#10556=ORIENTED_EDGE('',*,*,#8332,.T.);
#10557=ORIENTED_EDGE('',*,*,#8333,.F.);
#10558=ORIENTED_EDGE('',*,*,#8332,.F.);
#10559=ORIENTED_EDGE('',*,*,#8331,.T.);
#10560=ORIENTED_EDGE('',*,*,#8334,.F.);
#10561=ORIENTED_EDGE('',*,*,#8335,.T.);
#10562=ORIENTED_EDGE('',*,*,#8336,.F.);
#10563=ORIENTED_EDGE('',*,*,#8335,.F.);
#10564=ORIENTED_EDGE('',*,*,#8334,.T.);
#10565=ORIENTED_EDGE('',*,*,#8337,.F.);
#10566=ORIENTED_EDGE('',*,*,#8338,.T.);
#10567=ORIENTED_EDGE('',*,*,#8339,.T.);
#10568=ORIENTED_EDGE('',*,*,#8338,.F.);
#10569=ORIENTED_EDGE('',*,*,#8339,.F.);
#10570=ORIENTED_EDGE('',*,*,#8340,.F.);
#10571=ORIENTED_EDGE('',*,*,#8341,.T.);
#10572=ORIENTED_EDGE('',*,*,#8342,.T.);
#10573=ORIENTED_EDGE('',*,*,#8341,.F.);
#10574=ORIENTED_EDGE('',*,*,#8342,.F.);
#10575=ORIENTED_EDGE('',*,*,#8343,.F.);
#10576=ORIENTED_EDGE('',*,*,#8344,.F.);
#10577=ORIENTED_EDGE('',*,*,#8345,.F.);
#10578=ORIENTED_EDGE('',*,*,#8346,.F.);
#10579=ORIENTED_EDGE('',*,*,#8347,.F.);
#10580=ORIENTED_EDGE('',*,*,#8348,.F.);
#10581=ORIENTED_EDGE('',*,*,#8349,.F.);
#10582=ORIENTED_EDGE('',*,*,#8344,.T.);
#10583=ORIENTED_EDGE('',*,*,#8346,.T.);
#10584=ORIENTED_EDGE('',*,*,#8350,.F.);
#10585=ORIENTED_EDGE('',*,*,#8351,.F.);
#10586=ORIENTED_EDGE('',*,*,#8352,.T.);
#10587=ORIENTED_EDGE('',*,*,#8353,.F.);
#10588=ORIENTED_EDGE('',*,*,#8354,.T.);
#10589=ORIENTED_EDGE('',*,*,#8355,.T.);
#10590=ORIENTED_EDGE('',*,*,#8356,.T.);
#10591=ORIENTED_EDGE('',*,*,#8357,.T.);
#10592=ORIENTED_EDGE('',*,*,#8358,.F.);
#10593=ORIENTED_EDGE('',*,*,#8359,.T.);
#10594=ORIENTED_EDGE('',*,*,#8360,.F.);
#10595=ORIENTED_EDGE('',*,*,#8361,.T.);
#10596=ORIENTED_EDGE('',*,*,#8362,.F.);
#10597=ORIENTED_EDGE('',*,*,#8333,.T.);
#10598=ORIENTED_EDGE('',*,*,#8336,.T.);
#10599=ORIENTED_EDGE('',*,*,#8363,.T.);
#10600=ORIENTED_EDGE('',*,*,#8364,.T.);
#10601=ORIENTED_EDGE('',*,*,#8365,.T.);
#10602=ORIENTED_EDGE('',*,*,#8366,.T.);
#10603=ORIENTED_EDGE('',*,*,#8345,.T.);
#10604=ORIENTED_EDGE('',*,*,#8349,.T.);
#10605=ORIENTED_EDGE('',*,*,#8367,.T.);
#10606=ORIENTED_EDGE('',*,*,#8368,.T.);
#10607=ORIENTED_EDGE('',*,*,#8369,.T.);
#10608=ORIENTED_EDGE('',*,*,#8370,.T.);
#10609=ORIENTED_EDGE('',*,*,#8371,.T.);
#10610=ORIENTED_EDGE('',*,*,#8372,.T.);
#10611=ORIENTED_EDGE('',*,*,#8373,.T.);
#10612=ORIENTED_EDGE('',*,*,#8374,.T.);
#10613=ORIENTED_EDGE('',*,*,#8375,.T.);
#10614=ORIENTED_EDGE('',*,*,#8350,.T.);
#10615=ORIENTED_EDGE('',*,*,#8376,.T.);
#10616=ORIENTED_EDGE('',*,*,#8377,.T.);
#10617=ORIENTED_EDGE('',*,*,#8378,.T.);
#10618=ORIENTED_EDGE('',*,*,#8379,.T.);
#10619=ORIENTED_EDGE('',*,*,#8380,.T.);
#10620=ORIENTED_EDGE('',*,*,#8373,.F.);
#10621=ORIENTED_EDGE('',*,*,#8381,.T.);
#10622=ORIENTED_EDGE('',*,*,#8382,.F.);
#10623=ORIENTED_EDGE('',*,*,#8383,.F.);
#10624=ORIENTED_EDGE('',*,*,#8372,.F.);
#10625=ORIENTED_EDGE('',*,*,#8384,.F.);
#10626=ORIENTED_EDGE('',*,*,#8385,.F.);
#10627=ORIENTED_EDGE('',*,*,#8381,.F.);
#10628=ORIENTED_EDGE('',*,*,#8383,.T.);
#10629=ORIENTED_EDGE('',*,*,#8386,.F.);
#10630=ORIENTED_EDGE('',*,*,#8387,.T.);
#10631=ORIENTED_EDGE('',*,*,#8388,.F.);
#10632=ORIENTED_EDGE('',*,*,#8389,.T.);
#10633=ORIENTED_EDGE('',*,*,#8390,.F.);
#10634=ORIENTED_EDGE('',*,*,#8391,.F.);
#10635=ORIENTED_EDGE('',*,*,#8392,.T.);
#10636=ORIENTED_EDGE('',*,*,#8393,.F.);
#10637=ORIENTED_EDGE('',*,*,#8394,.T.);
#10638=ORIENTED_EDGE('',*,*,#8395,.T.);
#10639=ORIENTED_EDGE('',*,*,#8396,.T.);
#10640=ORIENTED_EDGE('',*,*,#8397,.T.);
#10641=ORIENTED_EDGE('',*,*,#8374,.F.);
#10642=ORIENTED_EDGE('',*,*,#8337,.T.);
#10643=ORIENTED_EDGE('',*,*,#8340,.T.);
#10644=ORIENTED_EDGE('',*,*,#8398,.T.);
#10645=ORIENTED_EDGE('',*,*,#8399,.T.);
#10646=ORIENTED_EDGE('',*,*,#8400,.T.);
#10647=ORIENTED_EDGE('',*,*,#8401,.T.);
#10648=ORIENTED_EDGE('',*,*,#8382,.T.);
#10649=ORIENTED_EDGE('',*,*,#8385,.T.);
#10650=ORIENTED_EDGE('',*,*,#8402,.T.);
#10651=ORIENTED_EDGE('',*,*,#8403,.T.);
#10652=ORIENTED_EDGE('',*,*,#8404,.T.);
#10653=ORIENTED_EDGE('',*,*,#8405,.T.);
#10654=ORIENTED_EDGE('',*,*,#8406,.T.);
#10655=ORIENTED_EDGE('',*,*,#8386,.T.);
#10656=ORIENTED_EDGE('',*,*,#8384,.T.);
#10657=ORIENTED_EDGE('',*,*,#8371,.F.);
#10658=ORIENTED_EDGE('',*,*,#8407,.F.);
#10659=ORIENTED_EDGE('',*,*,#8402,.F.);
#10660=ORIENTED_EDGE('',*,*,#8348,.T.);
#10661=ORIENTED_EDGE('',*,*,#8408,.F.);
#10662=ORIENTED_EDGE('',*,*,#8409,.F.);
#10663=ORIENTED_EDGE('',*,*,#8367,.F.);
#10664=ORIENTED_EDGE('',*,*,#8409,.T.);
#10665=ORIENTED_EDGE('',*,*,#8410,.F.);
#10666=ORIENTED_EDGE('',*,*,#8411,.T.);
#10667=ORIENTED_EDGE('',*,*,#8412,.F.);
#10668=ORIENTED_EDGE('',*,*,#8413,.T.);
#10669=ORIENTED_EDGE('',*,*,#8414,.F.);
#10670=ORIENTED_EDGE('',*,*,#8415,.F.);
#10671=ORIENTED_EDGE('',*,*,#8416,.F.);
#10672=ORIENTED_EDGE('',*,*,#8417,.T.);
#10673=ORIENTED_EDGE('',*,*,#8368,.F.);
#10674=ORIENTED_EDGE('',*,*,#8343,.T.);
#10675=ORIENTED_EDGE('',*,*,#8362,.T.);
#10676=ORIENTED_EDGE('',*,*,#8418,.T.);
#10677=ORIENTED_EDGE('',*,*,#8419,.T.);
#10678=ORIENTED_EDGE('',*,*,#8420,.T.);
#10679=ORIENTED_EDGE('',*,*,#8410,.T.);
#10680=ORIENTED_EDGE('',*,*,#8408,.T.);
#10681=ORIENTED_EDGE('',*,*,#8347,.T.);
#10682=ORIENTED_EDGE('',*,*,#8421,.F.);
#10683=ORIENTED_EDGE('',*,*,#8422,.T.);
#10684=ORIENTED_EDGE('',*,*,#8366,.F.);
#10685=ORIENTED_EDGE('',*,*,#8422,.F.);
#10686=ORIENTED_EDGE('',*,*,#8421,.T.);
#10687=ORIENTED_EDGE('',*,*,#8423,.F.);
#10688=ORIENTED_EDGE('',*,*,#8424,.T.);
#10689=ORIENTED_EDGE('',*,*,#8365,.F.);
#10690=ORIENTED_EDGE('',*,*,#8424,.F.);
#10691=ORIENTED_EDGE('',*,*,#8423,.T.);
#10692=ORIENTED_EDGE('',*,*,#8398,.F.);
#10693=ORIENTED_EDGE('',*,*,#8425,.T.);
#10694=ORIENTED_EDGE('',*,*,#8426,.T.);
#10695=ORIENTED_EDGE('',*,*,#8425,.F.);
#10696=ORIENTED_EDGE('',*,*,#8426,.F.);
#10697=ORIENTED_EDGE('',*,*,#8399,.F.);
#10698=ORIENTED_EDGE('',*,*,#8427,.T.);
#10699=ORIENTED_EDGE('',*,*,#8428,.T.);
#10700=ORIENTED_EDGE('',*,*,#8427,.F.);
#10701=ORIENTED_EDGE('',*,*,#8428,.F.);
#10702=ORIENTED_EDGE('',*,*,#8429,.F.);
#10703=ORIENTED_EDGE('',*,*,#8430,.F.);
#10704=ORIENTED_EDGE('',*,*,#8418,.F.);
#10705=ORIENTED_EDGE('',*,*,#8361,.F.);
#10706=ORIENTED_EDGE('',*,*,#8431,.F.);
#10707=ORIENTED_EDGE('',*,*,#8432,.F.);
#10708=ORIENTED_EDGE('',*,*,#8419,.F.);
#10709=ORIENTED_EDGE('',*,*,#8430,.T.);
#10710=ORIENTED_EDGE('',*,*,#8406,.F.);
#10711=ORIENTED_EDGE('',*,*,#8433,.T.);
#10712=ORIENTED_EDGE('',*,*,#8434,.F.);
#10713=ORIENTED_EDGE('',*,*,#8387,.F.);
#10714=ORIENTED_EDGE('',*,*,#8405,.F.);
#10715=ORIENTED_EDGE('',*,*,#8435,.F.);
#10716=ORIENTED_EDGE('',*,*,#8436,.F.);
#10717=ORIENTED_EDGE('',*,*,#8433,.F.);
#10718=ORIENTED_EDGE('',*,*,#8434,.T.);
#10719=ORIENTED_EDGE('',*,*,#8436,.T.);
#10720=ORIENTED_EDGE('',*,*,#8437,.T.);
#10721=ORIENTED_EDGE('',*,*,#8438,.T.);
#10722=ORIENTED_EDGE('',*,*,#8439,.T.);
#10723=ORIENTED_EDGE('',*,*,#8440,.T.);
#10724=ORIENTED_EDGE('',*,*,#8441,.T.);
#10725=ORIENTED_EDGE('',*,*,#8388,.T.);
#10726=ORIENTED_EDGE('',*,*,#8432,.T.);
#10727=ORIENTED_EDGE('',*,*,#8442,.F.);
#10728=ORIENTED_EDGE('',*,*,#8411,.F.);
#10729=ORIENTED_EDGE('',*,*,#8420,.F.);
#10730=ORIENTED_EDGE('',*,*,#8435,.T.);
#10731=ORIENTED_EDGE('',*,*,#8404,.F.);
#10732=ORIENTED_EDGE('',*,*,#8443,.F.);
#10733=ORIENTED_EDGE('',*,*,#8437,.F.);
#10734=ORIENTED_EDGE('',*,*,#8407,.T.);
#10735=ORIENTED_EDGE('',*,*,#8370,.F.);
#10736=ORIENTED_EDGE('',*,*,#8444,.F.);
#10737=ORIENTED_EDGE('',*,*,#8445,.F.);
#10738=ORIENTED_EDGE('',*,*,#8446,.T.);
#10739=ORIENTED_EDGE('',*,*,#8447,.F.);
#10740=ORIENTED_EDGE('',*,*,#8448,.T.);
#10741=ORIENTED_EDGE('',*,*,#8438,.F.);
#10742=ORIENTED_EDGE('',*,*,#8443,.T.);
#10743=ORIENTED_EDGE('',*,*,#8403,.F.);
#10744=ORIENTED_EDGE('',*,*,#8429,.T.);
#10745=ORIENTED_EDGE('',*,*,#8360,.T.);
#10746=ORIENTED_EDGE('',*,*,#8449,.T.);
#10747=ORIENTED_EDGE('',*,*,#8450,.T.);
#10748=ORIENTED_EDGE('',*,*,#8451,.T.);
#10749=ORIENTED_EDGE('',*,*,#8412,.T.);
#10750=ORIENTED_EDGE('',*,*,#8442,.T.);
#10751=ORIENTED_EDGE('',*,*,#8431,.T.);
#10752=ORIENTED_EDGE('',*,*,#8452,.F.);
#10753=ORIENTED_EDGE('',*,*,#8453,.T.);
#10754=ORIENTED_EDGE('',*,*,#8364,.F.);
#10755=ORIENTED_EDGE('',*,*,#8453,.F.);
#10756=ORIENTED_EDGE('',*,*,#8452,.T.);
#10757=ORIENTED_EDGE('',*,*,#8454,.F.);
#10758=ORIENTED_EDGE('',*,*,#8455,.T.);
#10759=ORIENTED_EDGE('',*,*,#8363,.F.);
#10760=ORIENTED_EDGE('',*,*,#8455,.F.);
#10761=ORIENTED_EDGE('',*,*,#8454,.T.);
#10762=ORIENTED_EDGE('',*,*,#8401,.F.);
#10763=ORIENTED_EDGE('',*,*,#8456,.T.);
#10764=ORIENTED_EDGE('',*,*,#8457,.T.);
#10765=ORIENTED_EDGE('',*,*,#8456,.F.);
#10766=ORIENTED_EDGE('',*,*,#8457,.F.);
#10767=ORIENTED_EDGE('',*,*,#8400,.F.);
#10768=ORIENTED_EDGE('',*,*,#8458,.T.);
#10769=ORIENTED_EDGE('',*,*,#8459,.T.);
#10770=ORIENTED_EDGE('',*,*,#8458,.F.);
#10771=ORIENTED_EDGE('',*,*,#8459,.F.);
#10772=ORIENTED_EDGE('',*,*,#8460,.F.);
#10773=ORIENTED_EDGE('',*,*,#8461,.F.);
#10774=ORIENTED_EDGE('',*,*,#8449,.F.);
#10775=ORIENTED_EDGE('',*,*,#8359,.F.);
#10776=ORIENTED_EDGE('',*,*,#8462,.F.);
#10777=ORIENTED_EDGE('',*,*,#8463,.F.);
#10778=ORIENTED_EDGE('',*,*,#8450,.F.);
#10779=ORIENTED_EDGE('',*,*,#8461,.T.);
#10780=ORIENTED_EDGE('',*,*,#8462,.T.);
#10781=ORIENTED_EDGE('',*,*,#8460,.T.);
#10782=ORIENTED_EDGE('',*,*,#8358,.T.);
#10783=ORIENTED_EDGE('',*,*,#8464,.T.);
#10784=ORIENTED_EDGE('',*,*,#8390,.T.);
#10785=ORIENTED_EDGE('',*,*,#8465,.T.);
#10786=ORIENTED_EDGE('',*,*,#8466,.T.);
#10787=ORIENTED_EDGE('',*,*,#8467,.T.);
#10788=ORIENTED_EDGE('',*,*,#8447,.T.);
#10789=ORIENTED_EDGE('',*,*,#8468,.T.);
#10790=ORIENTED_EDGE('',*,*,#8414,.T.);
#10791=ORIENTED_EDGE('',*,*,#8469,.T.);
#10792=ORIENTED_EDGE('',*,*,#8470,.T.);
#10793=ORIENTED_EDGE('',*,*,#8471,.T.);
#10794=ORIENTED_EDGE('',*,*,#8472,.T.);
#10795=ORIENTED_EDGE('',*,*,#8473,.T.);
#10796=ORIENTED_EDGE('',*,*,#8474,.T.);
#10797=ORIENTED_EDGE('',*,*,#8441,.F.);
#10798=ORIENTED_EDGE('',*,*,#8475,.T.);
#10799=ORIENTED_EDGE('',*,*,#8465,.F.);
#10800=ORIENTED_EDGE('',*,*,#8389,.F.);
#10801=ORIENTED_EDGE('',*,*,#8440,.F.);
#10802=ORIENTED_EDGE('',*,*,#8476,.F.);
#10803=ORIENTED_EDGE('',*,*,#8466,.F.);
#10804=ORIENTED_EDGE('',*,*,#8475,.F.);
#10805=ORIENTED_EDGE('',*,*,#8476,.T.);
#10806=ORIENTED_EDGE('',*,*,#8439,.F.);
#10807=ORIENTED_EDGE('',*,*,#8448,.F.);
#10808=ORIENTED_EDGE('',*,*,#8467,.F.);
#10809=ORIENTED_EDGE('',*,*,#8463,.T.);
#10810=ORIENTED_EDGE('',*,*,#8469,.F.);
#10811=ORIENTED_EDGE('',*,*,#8413,.F.);
#10812=ORIENTED_EDGE('',*,*,#8451,.F.);
#10813=ORIENTED_EDGE('',*,*,#8477,.F.);
#10814=ORIENTED_EDGE('',*,*,#8478,.T.);
#10815=ORIENTED_EDGE('',*,*,#8479,.F.);
#10816=ORIENTED_EDGE('',*,*,#8478,.F.);
#10817=ORIENTED_EDGE('',*,*,#8477,.T.);
#10818=ORIENTED_EDGE('',*,*,#8480,.F.);
#10819=ORIENTED_EDGE('',*,*,#8481,.F.);
#10820=ORIENTED_EDGE('',*,*,#8482,.T.);
#10821=ORIENTED_EDGE('',*,*,#8483,.F.);
#10822=ORIENTED_EDGE('',*,*,#8482,.F.);
#10823=ORIENTED_EDGE('',*,*,#8481,.T.);
#10824=ORIENTED_EDGE('',*,*,#8484,.F.);
#10825=ORIENTED_EDGE('',*,*,#8485,.F.);
#10826=ORIENTED_EDGE('',*,*,#8486,.T.);
#10827=ORIENTED_EDGE('',*,*,#8487,.F.);
#10828=ORIENTED_EDGE('',*,*,#8486,.F.);
#10829=ORIENTED_EDGE('',*,*,#8485,.T.);
#10830=ORIENTED_EDGE('',*,*,#8488,.F.);
#10831=ORIENTED_EDGE('',*,*,#8489,.F.);
#10832=ORIENTED_EDGE('',*,*,#8490,.T.);
#10833=ORIENTED_EDGE('',*,*,#8491,.F.);
#10834=ORIENTED_EDGE('',*,*,#8490,.F.);
#10835=ORIENTED_EDGE('',*,*,#8489,.T.);
#10836=ORIENTED_EDGE('',*,*,#8492,.F.);
#10837=ORIENTED_EDGE('',*,*,#8493,.F.);
#10838=ORIENTED_EDGE('',*,*,#8494,.T.);
#10839=ORIENTED_EDGE('',*,*,#8480,.T.);
#10840=ORIENTED_EDGE('',*,*,#8494,.F.);
#10841=ORIENTED_EDGE('',*,*,#8495,.F.);
#10842=ORIENTED_EDGE('',*,*,#8496,.T.);
#10843=ORIENTED_EDGE('',*,*,#8484,.T.);
#10844=ORIENTED_EDGE('',*,*,#8496,.F.);
#10845=ORIENTED_EDGE('',*,*,#8497,.F.);
#10846=ORIENTED_EDGE('',*,*,#8498,.T.);
#10847=ORIENTED_EDGE('',*,*,#8488,.T.);
#10848=ORIENTED_EDGE('',*,*,#8498,.F.);
#10849=ORIENTED_EDGE('',*,*,#8499,.F.);
#10850=ORIENTED_EDGE('',*,*,#8500,.T.);
#10851=ORIENTED_EDGE('',*,*,#8492,.T.);
#10852=ORIENTED_EDGE('',*,*,#8500,.F.);
#10853=ORIENTED_EDGE('',*,*,#8501,.F.);
#10854=ORIENTED_EDGE('',*,*,#8502,.T.);
#10855=ORIENTED_EDGE('',*,*,#8376,.F.);
#10856=ORIENTED_EDGE('',*,*,#8502,.F.);
#10857=ORIENTED_EDGE('',*,*,#8501,.T.);
#10858=ORIENTED_EDGE('',*,*,#8503,.F.);
#10859=ORIENTED_EDGE('',*,*,#8504,.T.);
#10860=ORIENTED_EDGE('',*,*,#8380,.F.);
#10861=ORIENTED_EDGE('',*,*,#8504,.F.);
#10862=ORIENTED_EDGE('',*,*,#8503,.T.);
#10863=ORIENTED_EDGE('',*,*,#8505,.F.);
#10864=ORIENTED_EDGE('',*,*,#8506,.T.);
#10865=ORIENTED_EDGE('',*,*,#8470,.F.);
#10866=ORIENTED_EDGE('',*,*,#8506,.F.);
#10867=ORIENTED_EDGE('',*,*,#8505,.T.);
#10868=ORIENTED_EDGE('',*,*,#8507,.F.);
#10869=ORIENTED_EDGE('',*,*,#8508,.T.);
#10870=ORIENTED_EDGE('',*,*,#8474,.F.);
#10871=ORIENTED_EDGE('',*,*,#8508,.F.);
#10872=ORIENTED_EDGE('',*,*,#8507,.T.);
#10873=ORIENTED_EDGE('',*,*,#8509,.F.);
#10874=ORIENTED_EDGE('',*,*,#8510,.T.);
#10875=ORIENTED_EDGE('',*,*,#8377,.F.);
#10876=ORIENTED_EDGE('',*,*,#8510,.F.);
#10877=ORIENTED_EDGE('',*,*,#8511,.F.);
#10878=ORIENTED_EDGE('',*,*,#8512,.T.);
#10879=ORIENTED_EDGE('',*,*,#8471,.F.);
#10880=ORIENTED_EDGE('',*,*,#8512,.F.);
#10881=ORIENTED_EDGE('',*,*,#8513,.F.);
#10882=ORIENTED_EDGE('',*,*,#8514,.T.);
#10883=ORIENTED_EDGE('',*,*,#8472,.F.);
#10884=ORIENTED_EDGE('',*,*,#8514,.F.);
#10885=ORIENTED_EDGE('',*,*,#8515,.F.);
#10886=ORIENTED_EDGE('',*,*,#8516,.T.);
#10887=ORIENTED_EDGE('',*,*,#8473,.F.);
#10888=ORIENTED_EDGE('',*,*,#8516,.F.);
#10889=ORIENTED_EDGE('',*,*,#8517,.F.);
#10890=ORIENTED_EDGE('',*,*,#8518,.T.);
#10891=ORIENTED_EDGE('',*,*,#8378,.F.);
#10892=ORIENTED_EDGE('',*,*,#8518,.F.);
#10893=ORIENTED_EDGE('',*,*,#8519,.F.);
#10894=ORIENTED_EDGE('',*,*,#8520,.T.);
#10895=ORIENTED_EDGE('',*,*,#8379,.F.);
#10896=ORIENTED_EDGE('',*,*,#8520,.F.);
#10897=ORIENTED_EDGE('',*,*,#8521,.T.);
#10898=ORIENTED_EDGE('',*,*,#8351,.T.);
#10899=ORIENTED_EDGE('',*,*,#8375,.F.);
#10900=ORIENTED_EDGE('',*,*,#8397,.F.);
#10901=ORIENTED_EDGE('',*,*,#8522,.F.);
#10902=ORIENTED_EDGE('',*,*,#8352,.F.);
#10903=ORIENTED_EDGE('',*,*,#8521,.F.);
#10904=ORIENTED_EDGE('',*,*,#8396,.F.);
#10905=ORIENTED_EDGE('',*,*,#8509,.T.);
#10906=ORIENTED_EDGE('',*,*,#8517,.T.);
#10907=ORIENTED_EDGE('',*,*,#8519,.T.);
#10908=ORIENTED_EDGE('',*,*,#8522,.T.);
#10909=ORIENTED_EDGE('',*,*,#8395,.F.);
#10910=ORIENTED_EDGE('',*,*,#8523,.T.);
#10911=ORIENTED_EDGE('',*,*,#8353,.T.);
#10912=ORIENTED_EDGE('',*,*,#8524,.T.);
#10913=ORIENTED_EDGE('',*,*,#8391,.T.);
#10914=ORIENTED_EDGE('',*,*,#8464,.F.);
#10915=ORIENTED_EDGE('',*,*,#8357,.F.);
#10916=ORIENTED_EDGE('',*,*,#8524,.F.);
#10917=ORIENTED_EDGE('',*,*,#8356,.F.);
#10918=ORIENTED_EDGE('',*,*,#8525,.F.);
#10919=ORIENTED_EDGE('',*,*,#8392,.F.);
#10920=ORIENTED_EDGE('',*,*,#8511,.T.);
#10921=ORIENTED_EDGE('',*,*,#8513,.T.);
#10922=ORIENTED_EDGE('',*,*,#8515,.T.);
#10923=ORIENTED_EDGE('',*,*,#8468,.F.);
#10924=ORIENTED_EDGE('',*,*,#8446,.F.);
#10925=ORIENTED_EDGE('',*,*,#8526,.F.);
#10926=ORIENTED_EDGE('',*,*,#8415,.T.);
#10927=ORIENTED_EDGE('',*,*,#8369,.F.);
#10928=ORIENTED_EDGE('',*,*,#8417,.F.);
#10929=ORIENTED_EDGE('',*,*,#8527,.F.);
#10930=ORIENTED_EDGE('',*,*,#8444,.T.);
#10931=ORIENTED_EDGE('',*,*,#8526,.T.);
#10932=ORIENTED_EDGE('',*,*,#8445,.T.);
#10933=ORIENTED_EDGE('',*,*,#8527,.T.);
#10934=ORIENTED_EDGE('',*,*,#8416,.T.);
#10935=ORIENTED_EDGE('',*,*,#8491,.T.);
#10936=ORIENTED_EDGE('',*,*,#8487,.T.);
#10937=ORIENTED_EDGE('',*,*,#8483,.T.);
#10938=ORIENTED_EDGE('',*,*,#8479,.T.);
#10939=ORIENTED_EDGE('',*,*,#8525,.T.);
#10940=ORIENTED_EDGE('',*,*,#8355,.F.);
#10941=ORIENTED_EDGE('',*,*,#8528,.T.);
#10942=ORIENTED_EDGE('',*,*,#8393,.T.);
#10943=ORIENTED_EDGE('',*,*,#8528,.F.);
#10944=ORIENTED_EDGE('',*,*,#8354,.F.);
#10945=ORIENTED_EDGE('',*,*,#8523,.F.);
#10946=ORIENTED_EDGE('',*,*,#8394,.F.);
#10947=ORIENTED_EDGE('',*,*,#8493,.T.);
#10948=ORIENTED_EDGE('',*,*,#8495,.T.);
#10949=ORIENTED_EDGE('',*,*,#8497,.T.);
#10950=ORIENTED_EDGE('',*,*,#8499,.T.);
#14911=CYLINDRICAL_SURFACE('',#16834,0.164999999999999);
#14912=CYLINDRICAL_SURFACE('',#16838,0.164999999999999);
#14913=CYLINDRICAL_SURFACE('',#16842,0.164999999999999);
#14914=CYLINDRICAL_SURFACE('',#16846,0.164999999999999);
#14915=CYLINDRICAL_SURFACE('',#16850,2.35);
#14916=CYLINDRICAL_SURFACE('',#16868,2.35);
#14917=CYLINDRICAL_SURFACE('',#16881,1.9);
#14918=CYLINDRICAL_SURFACE('',#16883,1.9);
#14919=CYLINDRICAL_SURFACE('',#16889,0.165);
#14920=CYLINDRICAL_SURFACE('',#16892,0.165);
#14921=CYLINDRICAL_SURFACE('',#16895,0.165);
#14922=CYLINDRICAL_SURFACE('',#16898,0.165);
#14923=CYLINDRICAL_SURFACE('',#16901,2.35);
#14924=CYLINDRICAL_SURFACE('',#16905,2.35);
#14925=CYLINDRICAL_SURFACE('',#16910,1.9);
#14926=CYLINDRICAL_SURFACE('',#16911,1.9);
#14927=CYLINDRICAL_SURFACE('',#16916,0.165);
#14928=CYLINDRICAL_SURFACE('',#16919,0.165);
#14929=CYLINDRICAL_SURFACE('',#16922,0.165);
#14930=CYLINDRICAL_SURFACE('',#16925,0.165);
#14931=CYLINDRICAL_SURFACE('',#16928,1.6);
#14932=CYLINDRICAL_SURFACE('',#16938,1.6);
#14933=CYLINDRICAL_SURFACE('',#16942,1.2);
#14934=CYLINDRICAL_SURFACE('',#16943,1.2);
#14935=CYLINDRICAL_SURFACE('',#16944,0.6);
#14936=CYLINDRICAL_SURFACE('',#16949,0.6);
#14937=CYLINDRICAL_SURFACE('',#16954,0.6);
#14938=CYLINDRICAL_SURFACE('',#16959,0.6);
#14939=CYLINDRICAL_SURFACE('',#16964,0.33);
#14940=CYLINDRICAL_SURFACE('',#16966,0.33);
#14941=CYLINDRICAL_SURFACE('',#16968,0.33);
#14942=CYLINDRICAL_SURFACE('',#16970,0.33);
#14943=CYLINDRICAL_SURFACE('',#16972,0.149999999999999);
#14944=CYLINDRICAL_SURFACE('',#16975,0.149999999999999);
#14945=CYLINDRICAL_SURFACE('',#16978,0.15);
#14946=CYLINDRICAL_SURFACE('',#16981,0.15);
#14947=CYLINDRICAL_SURFACE('',#16984,0.25);
#14948=CYLINDRICAL_SURFACE('',#16986,0.25);
#14949=CYLINDRICAL_SURFACE('',#16988,0.25);
#14950=CYLINDRICAL_SURFACE('',#16990,0.25);
#14951=CYLINDRICAL_SURFACE('',#16992,0.25);
#14952=CYLINDRICAL_SURFACE('',#16994,0.25);
#15219=ADVANCED_FACE('',(#2012),#14911,.F.);
#15220=ADVANCED_FACE('',(#2013),#1608,.T.);
#15221=ADVANCED_FACE('',(#2014),#14912,.F.);
#15222=ADVANCED_FACE('',(#2015),#1609,.T.);
#15223=ADVANCED_FACE('',(#2016),#14913,.F.);
#15224=ADVANCED_FACE('',(#2017),#1610,.F.);
#15225=ADVANCED_FACE('',(#2018),#14914,.F.);
#15226=ADVANCED_FACE('',(#2019),#1611,.F.);
#15227=ADVANCED_FACE('',(#2020),#14915,.F.);
#15228=ADVANCED_FACE('',(#2021),#1612,.T.);
#15229=ADVANCED_FACE('',(#2022,#1382,#1383,#1384,#1385,#1386,#1387),#1613,
 .T.);
#15230=ADVANCED_FACE('',(#2023,#1388,#1389,#1390,#1391,#1392),#1614,.T.);
#15231=ADVANCED_FACE('',(#2024),#14916,.F.);
#15232=ADVANCED_FACE('',(#2025),#1615,.F.);
#15233=ADVANCED_FACE('',(#2026,#1393,#1394,#1395,#1396,#1397,#1398),#1616,
 .T.);
#15234=ADVANCED_FACE('',(#2027),#1617,.T.);
#15235=ADVANCED_FACE('',(#2028),#14917,.F.);
#15236=ADVANCED_FACE('',(#2029),#14918,.F.);
#15237=ADVANCED_FACE('',(#2030),#1618,.F.);
#15238=ADVANCED_FACE('',(#2031),#1619,.T.);
#15239=ADVANCED_FACE('',(#2032),#14919,.F.);
#15240=ADVANCED_FACE('',(#2033),#1620,.T.);
#15241=ADVANCED_FACE('',(#2034),#14920,.F.);
#15242=ADVANCED_FACE('',(#2035),#1621,.T.);
#15243=ADVANCED_FACE('',(#2036),#14921,.F.);
#15244=ADVANCED_FACE('',(#2037),#1622,.F.);
#15245=ADVANCED_FACE('',(#2038),#14922,.F.);
#15246=ADVANCED_FACE('',(#2039),#1623,.F.);
#15247=ADVANCED_FACE('',(#2040),#14923,.F.);
#15248=ADVANCED_FACE('',(#2041),#1624,.T.);
#15249=ADVANCED_FACE('',(#2042),#14924,.F.);
#15250=ADVANCED_FACE('',(#2043),#1625,.F.);
#15251=ADVANCED_FACE('',(#2044),#1626,.T.);
#15252=ADVANCED_FACE('',(#2045),#14925,.F.);
#15253=ADVANCED_FACE('',(#2046),#14926,.F.);
#15254=ADVANCED_FACE('',(#2047),#1627,.F.);
#15255=ADVANCED_FACE('',(#2048),#1628,.T.);
#15256=ADVANCED_FACE('',(#2049),#14927,.F.);
#15257=ADVANCED_FACE('',(#2050),#1629,.T.);
#15258=ADVANCED_FACE('',(#2051),#14928,.F.);
#15259=ADVANCED_FACE('',(#2052),#1630,.T.);
#15260=ADVANCED_FACE('',(#2053),#14929,.F.);
#15261=ADVANCED_FACE('',(#2054),#1631,.F.);
#15262=ADVANCED_FACE('',(#2055),#14930,.F.);
#15263=ADVANCED_FACE('',(#2056),#1632,.F.);
#15264=ADVANCED_FACE('',(#2057),#14931,.F.);
#15265=ADVANCED_FACE('',(#2058),#1633,.T.);
#15266=ADVANCED_FACE('',(#2059,#1399,#1400,#1401,#1402,#1403),#1634,.T.);
#15267=ADVANCED_FACE('',(#2060),#14932,.F.);
#15268=ADVANCED_FACE('',(#2061),#1635,.F.);
#15269=ADVANCED_FACE('',(#2062),#14933,.F.);
#15270=ADVANCED_FACE('',(#2063),#14934,.F.);
#15271=ADVANCED_FACE('',(#2064),#14935,.F.);
#15272=ADVANCED_FACE('',(#2065,#1404),#1636,.T.);
#15273=ADVANCED_FACE('',(#2066),#14936,.F.);
#15274=ADVANCED_FACE('',(#2067,#1405),#1637,.T.);
#15275=ADVANCED_FACE('',(#2068),#14937,.F.);
#15276=ADVANCED_FACE('',(#2069,#1406),#1638,.T.);
#15277=ADVANCED_FACE('',(#2070),#14938,.F.);
#15278=ADVANCED_FACE('',(#2071,#1407),#1639,.T.);
#15279=ADVANCED_FACE('',(#2072),#14939,.F.);
#15280=ADVANCED_FACE('',(#2073),#14940,.F.);
#15281=ADVANCED_FACE('',(#2074),#14941,.F.);
#15282=ADVANCED_FACE('',(#2075),#14942,.F.);
#15283=ADVANCED_FACE('',(#2076),#14943,.F.);
#15284=ADVANCED_FACE('',(#2077),#1640,.T.);
#15285=ADVANCED_FACE('',(#2078),#14944,.F.);
#15286=ADVANCED_FACE('',(#2079),#1641,.T.);
#15287=ADVANCED_FACE('',(#2080),#14945,.F.);
#15288=ADVANCED_FACE('',(#2081),#1642,.T.);
#15289=ADVANCED_FACE('',(#2082),#14946,.F.);
#15290=ADVANCED_FACE('',(#2083),#1643,.T.);
#15291=ADVANCED_FACE('',(#2084),#14947,.F.);
#15292=ADVANCED_FACE('',(#2085),#14948,.F.);
#15293=ADVANCED_FACE('',(#2086),#14949,.F.);
#15294=ADVANCED_FACE('',(#2087),#14950,.F.);
#15295=ADVANCED_FACE('',(#2088),#14951,.F.);
#15296=ADVANCED_FACE('',(#2089),#14952,.F.);
#15297=ADVANCED_FACE('',(#2090),#1644,.T.);
#15298=ADVANCED_FACE('',(#2091,#1408,#1409,#1410),#1645,.F.);
#15299=ADVANCED_FACE('',(#2092),#1646,.T.);
#15300=ADVANCED_FACE('',(#2093),#1647,.T.);
#15301=ADVANCED_FACE('',(#2094,#1411,#1412,#1413),#1648,.F.);
#15302=ADVANCED_FACE('',(#2095),#1649,.F.);
#15303=ADVANCED_FACE('',(#2096),#1650,.F.);
#15304=ADVANCED_FACE('',(#2097,#1414,#1415,#1416,#1417),#1651,.T.);
#15305=ADVANCED_FACE('',(#2098),#1652,.T.);
#15306=ADVANCED_FACE('',(#2099,#1418,#1419,#1420,#1421),#1653,.F.);
#16123=CLOSED_SHELL('',(#15219,#15220,#15221,#15222,#15223,#15224,#15225,
#15226,#15227,#15228,#15229,#15230,#15231,#15232,#15233,#15234,#15235,#15236,
#15237,#15238,#15239,#15240,#15241,#15242,#15243,#15244,#15245,#15246,#15247,
#15248,#15249,#15250,#15251,#15252,#15253,#15254,#15255,#15256,#15257,#15258,
#15259,#15260,#15261,#15262,#15263,#15264,#15265,#15266,#15267,#15268,#15269,
#15270,#15271,#15272,#15273,#15274,#15275,#15276,#15277,#15278,#15279,#15280,
#15281,#15282,#15283,#15284,#15285,#15286,#15287,#15288,#15289,#15290,#15291,
#15292,#15293,#15294,#15295,#15296,#15297,#15298,#15299,#15300,#15301,#15302,
#15303,#15304,#15305,#15306));
#16833=AXIS2_PLACEMENT_3D('',#22827,#18516,#18517);
#16834=AXIS2_PLACEMENT_3D('',#22828,#18518,#18519);
#16835=AXIS2_PLACEMENT_3D('',#22830,#18520,#18521);
#16836=AXIS2_PLACEMENT_3D('',#22833,#18523,#18524);
#16837=AXIS2_PLACEMENT_3D('',#22834,#18525,#18526);
#16838=AXIS2_PLACEMENT_3D('',#22835,#18527,#18528);
#16839=AXIS2_PLACEMENT_3D('',#22837,#18529,#18530);
#16840=AXIS2_PLACEMENT_3D('',#22840,#18532,#18533);
#16841=AXIS2_PLACEMENT_3D('',#22841,#18534,#18535);
#16842=AXIS2_PLACEMENT_3D('',#22842,#18536,#18537);
#16843=AXIS2_PLACEMENT_3D('',#22844,#18538,#18539);
#16844=AXIS2_PLACEMENT_3D('',#22847,#18541,#18542);
#16845=AXIS2_PLACEMENT_3D('',#22848,#18543,#18544);
#16846=AXIS2_PLACEMENT_3D('',#22849,#18545,#18546);
#16847=AXIS2_PLACEMENT_3D('',#22851,#18547,#18548);
#16848=AXIS2_PLACEMENT_3D('',#22854,#18550,#18551);
#16849=AXIS2_PLACEMENT_3D('',#22855,#18552,#18553);
#16850=AXIS2_PLACEMENT_3D('',#22856,#18554,#18555);
#16851=AXIS2_PLACEMENT_3D('',#22861,#18557,#18558);
#16852=AXIS2_PLACEMENT_3D('',#22864,#18560,#18561);
#16853=AXIS2_PLACEMENT_3D('',#22865,#18562,#18563);
#16854=AXIS2_PLACEMENT_3D('',#22869,#18565,#18566);
#16855=AXIS2_PLACEMENT_3D('',#22871,#18568,#18569);
#16856=AXIS2_PLACEMENT_3D('',#22891,#18579,#18580);
#16857=AXIS2_PLACEMENT_3D('',#22895,#18582,#18583);
#16858=AXIS2_PLACEMENT_3D('',#22898,#18585,#18586);
#16859=AXIS2_PLACEMENT_3D('',#22900,#18587,#18588);
#16860=AXIS2_PLACEMENT_3D('',#22902,#18589,#18590);
#16861=AXIS2_PLACEMENT_3D('',#22904,#18591,#18592);
#16862=AXIS2_PLACEMENT_3D('',#22905,#18593,#18594);
#16863=AXIS2_PLACEMENT_3D('',#22924,#18604,#18605);
#16864=AXIS2_PLACEMENT_3D('',#22926,#18606,#18607);
#16865=AXIS2_PLACEMENT_3D('',#22928,#18608,#18609);
#16866=AXIS2_PLACEMENT_3D('',#22930,#18610,#18611);
#16867=AXIS2_PLACEMENT_3D('',#22932,#18612,#18613);
#16868=AXIS2_PLACEMENT_3D('',#22933,#18614,#18615);
#16869=AXIS2_PLACEMENT_3D('',#22935,#18616,#18617);
#16870=AXIS2_PLACEMENT_3D('',#22938,#18619,#18620);
#16871=AXIS2_PLACEMENT_3D('',#22939,#18621,#18622);
#16872=AXIS2_PLACEMENT_3D('',#22941,#18623,#18624);
#16873=AXIS2_PLACEMENT_3D('',#22943,#18626,#18627);
#16874=AXIS2_PLACEMENT_3D('',#22947,#18629,#18630);
#16875=AXIS2_PLACEMENT_3D('',#22951,#18632,#18633);
#16876=AXIS2_PLACEMENT_3D('',#22968,#18642,#18643);
#16877=AXIS2_PLACEMENT_3D('',#22970,#18644,#18645);
#16878=AXIS2_PLACEMENT_3D('',#22972,#18646,#18647);
#16879=AXIS2_PLACEMENT_3D('',#22974,#18648,#18649);
#16880=AXIS2_PLACEMENT_3D('',#22975,#18650,#18651);
#16881=AXIS2_PLACEMENT_3D('',#22985,#18657,#18658);
#16882=AXIS2_PLACEMENT_3D('',#22986,#18659,#18660);
#16883=AXIS2_PLACEMENT_3D('',#22987,#18661,#18662);
#16884=AXIS2_PLACEMENT_3D('',#22990,#18664,#18665);
#16885=AXIS2_PLACEMENT_3D('',#22991,#18666,#18667);
#16886=AXIS2_PLACEMENT_3D('',#22995,#18669,#18670);
#16887=AXIS2_PLACEMENT_3D('',#22999,#18672,#18673);
#16888=AXIS2_PLACEMENT_3D('',#23007,#18678,#18679);
#16889=AXIS2_PLACEMENT_3D('',#23013,#18683,#18684);
#16890=AXIS2_PLACEMENT_3D('',#23015,#18685,#18686);
#16891=AXIS2_PLACEMENT_3D('',#23017,#18688,#18689);
#16892=AXIS2_PLACEMENT_3D('',#23018,#18690,#18691);
#16893=AXIS2_PLACEMENT_3D('',#23020,#18692,#18693);
#16894=AXIS2_PLACEMENT_3D('',#23022,#18695,#18696);
#16895=AXIS2_PLACEMENT_3D('',#23023,#18697,#18698);
#16896=AXIS2_PLACEMENT_3D('',#23026,#18700,#18701);
#16897=AXIS2_PLACEMENT_3D('',#23027,#18702,#18703);
#16898=AXIS2_PLACEMENT_3D('',#23028,#18704,#18705);
#16899=AXIS2_PLACEMENT_3D('',#23031,#18707,#18708);
#16900=AXIS2_PLACEMENT_3D('',#23032,#18709,#18710);
#16901=AXIS2_PLACEMENT_3D('',#23033,#18711,#18712);
#16902=AXIS2_PLACEMENT_3D('',#23036,#18714,#18715);
#16903=AXIS2_PLACEMENT_3D('',#23037,#18716,#18717);
#16904=AXIS2_PLACEMENT_3D('',#23040,#18719,#18720);
#16905=AXIS2_PLACEMENT_3D('',#23041,#18721,#18722);
#16906=AXIS2_PLACEMENT_3D('',#23043,#18723,#18724);
#16907=AXIS2_PLACEMENT_3D('',#23045,#18726,#18727);
#16908=AXIS2_PLACEMENT_3D('',#23047,#18728,#18729);
#16909=AXIS2_PLACEMENT_3D('',#23049,#18731,#18732);
#16910=AXIS2_PLACEMENT_3D('',#23059,#18738,#18739);
#16911=AXIS2_PLACEMENT_3D('',#23061,#18741,#18742);
#16912=AXIS2_PLACEMENT_3D('',#23062,#18743,#18744);
#16913=AXIS2_PLACEMENT_3D('',#23063,#18745,#18746);
#16914=AXIS2_PLACEMENT_3D('',#23072,#18751,#18752);
#16915=AXIS2_PLACEMENT_3D('',#23073,#18753,#18754);
#16916=AXIS2_PLACEMENT_3D('',#23079,#18758,#18759);
#16917=AXIS2_PLACEMENT_3D('',#23081,#18760,#18761);
#16918=AXIS2_PLACEMENT_3D('',#23083,#18763,#18764);
#16919=AXIS2_PLACEMENT_3D('',#23084,#18765,#18766);
#16920=AXIS2_PLACEMENT_3D('',#23086,#18767,#18768);
#16921=AXIS2_PLACEMENT_3D('',#23088,#18770,#18771);
#16922=AXIS2_PLACEMENT_3D('',#23089,#18772,#18773);
#16923=AXIS2_PLACEMENT_3D('',#23092,#18775,#18776);
#16924=AXIS2_PLACEMENT_3D('',#23093,#18777,#18778);
#16925=AXIS2_PLACEMENT_3D('',#23094,#18779,#18780);
#16926=AXIS2_PLACEMENT_3D('',#23097,#18782,#18783);
#16927=AXIS2_PLACEMENT_3D('',#23098,#18784,#18785);
#16928=AXIS2_PLACEMENT_3D('',#23099,#18786,#18787);
#16929=AXIS2_PLACEMENT_3D('',#23102,#18789,#18790);
#16930=AXIS2_PLACEMENT_3D('',#23103,#18791,#18792);
#16931=AXIS2_PLACEMENT_3D('',#23106,#18794,#18795);
#16932=AXIS2_PLACEMENT_3D('',#23107,#18796,#18797);
#16933=AXIS2_PLACEMENT_3D('',#23117,#18804,#18805);
#16934=AXIS2_PLACEMENT_3D('',#23119,#18806,#18807);
#16935=AXIS2_PLACEMENT_3D('',#23121,#18808,#18809);
#16936=AXIS2_PLACEMENT_3D('',#23123,#18810,#18811);
#16937=AXIS2_PLACEMENT_3D('',#23125,#18812,#18813);
#16938=AXIS2_PLACEMENT_3D('',#23126,#18814,#18815);
#16939=AXIS2_PLACEMENT_3D('',#23127,#18816,#18817);
#16940=AXIS2_PLACEMENT_3D('',#23128,#18818,#18819);
#16941=AXIS2_PLACEMENT_3D('',#23129,#18820,#18821);
#16942=AXIS2_PLACEMENT_3D('',#23130,#18822,#18823);
#16943=AXIS2_PLACEMENT_3D('',#23131,#18824,#18825);
#16944=AXIS2_PLACEMENT_3D('',#23132,#18826,#18827);
#16945=AXIS2_PLACEMENT_3D('',#23134,#18828,#18829);
#16946=AXIS2_PLACEMENT_3D('',#23137,#18831,#18832);
#16947=AXIS2_PLACEMENT_3D('',#23138,#18833,#18834);
#16948=AXIS2_PLACEMENT_3D('',#23140,#18835,#18836);
#16949=AXIS2_PLACEMENT_3D('',#23141,#18837,#18838);
#16950=AXIS2_PLACEMENT_3D('',#23143,#18839,#18840);
#16951=AXIS2_PLACEMENT_3D('',#23146,#18842,#18843);
#16952=AXIS2_PLACEMENT_3D('',#23147,#18844,#18845);
#16953=AXIS2_PLACEMENT_3D('',#23149,#18846,#18847);
#16954=AXIS2_PLACEMENT_3D('',#23150,#18848,#18849);
#16955=AXIS2_PLACEMENT_3D('',#23152,#18850,#18851);
#16956=AXIS2_PLACEMENT_3D('',#23155,#18853,#18854);
#16957=AXIS2_PLACEMENT_3D('',#23156,#18855,#18856);
#16958=AXIS2_PLACEMENT_3D('',#23158,#18857,#18858);
#16959=AXIS2_PLACEMENT_3D('',#23159,#18859,#18860);
#16960=AXIS2_PLACEMENT_3D('',#23161,#18861,#18862);
#16961=AXIS2_PLACEMENT_3D('',#23164,#18864,#18865);
#16962=AXIS2_PLACEMENT_3D('',#23165,#18866,#18867);
#16963=AXIS2_PLACEMENT_3D('',#23167,#18868,#18869);
#16964=AXIS2_PLACEMENT_3D('',#23168,#18870,#18871);
#16965=AXIS2_PLACEMENT_3D('',#23170,#18872,#18873);
#16966=AXIS2_PLACEMENT_3D('',#23172,#18875,#18876);
#16967=AXIS2_PLACEMENT_3D('',#23174,#18877,#18878);
#16968=AXIS2_PLACEMENT_3D('',#23176,#18880,#18881);
#16969=AXIS2_PLACEMENT_3D('',#23178,#18882,#18883);
#16970=AXIS2_PLACEMENT_3D('',#23180,#18885,#18886);
#16971=AXIS2_PLACEMENT_3D('',#23182,#18887,#18888);
#16972=AXIS2_PLACEMENT_3D('',#23184,#18890,#18891);
#16973=AXIS2_PLACEMENT_3D('',#23186,#18892,#18893);
#16974=AXIS2_PLACEMENT_3D('',#23188,#18895,#18896);
#16975=AXIS2_PLACEMENT_3D('',#23189,#18897,#18898);
#16976=AXIS2_PLACEMENT_3D('',#23191,#18899,#18900);
#16977=AXIS2_PLACEMENT_3D('',#23193,#18902,#18903);
#16978=AXIS2_PLACEMENT_3D('',#23194,#18904,#18905);
#16979=AXIS2_PLACEMENT_3D('',#23196,#18906,#18907);
#16980=AXIS2_PLACEMENT_3D('',#23198,#18909,#18910);
#16981=AXIS2_PLACEMENT_3D('',#23199,#18911,#18912);
#16982=AXIS2_PLACEMENT_3D('',#23201,#18913,#18914);
#16983=AXIS2_PLACEMENT_3D('',#23203,#18916,#18917);
#16984=AXIS2_PLACEMENT_3D('',#23204,#18918,#18919);
#16985=AXIS2_PLACEMENT_3D('',#23206,#18920,#18921);
#16986=AXIS2_PLACEMENT_3D('',#23208,#18923,#18924);
#16987=AXIS2_PLACEMENT_3D('',#23210,#18925,#18926);
#16988=AXIS2_PLACEMENT_3D('',#23212,#18928,#18929);
#16989=AXIS2_PLACEMENT_3D('',#23214,#18930,#18931);
#16990=AXIS2_PLACEMENT_3D('',#23216,#18933,#18934);
#16991=AXIS2_PLACEMENT_3D('',#23218,#18935,#18936);
#16992=AXIS2_PLACEMENT_3D('',#23220,#18938,#18939);
#16993=AXIS2_PLACEMENT_3D('',#23222,#18940,#18941);
#16994=AXIS2_PLACEMENT_3D('',#23224,#18943,#18944);
#16995=AXIS2_PLACEMENT_3D('',#23226,#18945,#18946);
#16996=AXIS2_PLACEMENT_3D('',#23228,#18948,#18949);
#16997=AXIS2_PLACEMENT_3D('',#23230,#18951,#18952);
#16998=AXIS2_PLACEMENT_3D('',#23232,#18954,#18955);
#16999=AXIS2_PLACEMENT_3D('',#23234,#18957,#18958);
#17000=AXIS2_PLACEMENT_3D('',#23236,#18960,#18961);
#17001=AXIS2_PLACEMENT_3D('',#23238,#18963,#18964);
#17002=AXIS2_PLACEMENT_3D('',#23240,#18966,#18967);
#17003=AXIS2_PLACEMENT_3D('',#23242,#18969,#18970);
#17004=AXIS2_PLACEMENT_3D('',#23243,#18971,#18972);
#17005=AXIS2_PLACEMENT_3D('',#23245,#18974,#18975);
#18516=DIRECTION('axis',(0.,0.,1.));
#18517=DIRECTION('refdir',(1.,0.,0.));
#18518=DIRECTION('center_axis',(0.,1.,0.));
#18519=DIRECTION('ref_axis',(1.,0.,0.));
#18520=DIRECTION('center_axis',(0.,1.,0.));
#18521=DIRECTION('ref_axis',(1.,0.,0.));
#18522=DIRECTION('',(0.,1.,0.));
#18523=DIRECTION('center_axis',(0.,-1.,0.));
#18524=DIRECTION('ref_axis',(1.,0.,0.));
#18525=DIRECTION('center_axis',(0.,1.,0.));
#18526=DIRECTION('ref_axis',(1.,0.,0.));
#18527=DIRECTION('center_axis',(0.,1.,0.));
#18528=DIRECTION('ref_axis',(1.,0.,0.));
#18529=DIRECTION('center_axis',(0.,1.,0.));
#18530=DIRECTION('ref_axis',(1.,0.,0.));
#18531=DIRECTION('',(0.,1.,0.));
#18532=DIRECTION('center_axis',(0.,-1.,0.));
#18533=DIRECTION('ref_axis',(1.,0.,0.));
#18534=DIRECTION('center_axis',(0.,1.,0.));
#18535=DIRECTION('ref_axis',(1.,0.,0.));
#18536=DIRECTION('center_axis',(0.,1.,0.));
#18537=DIRECTION('ref_axis',(1.,0.,0.));
#18538=DIRECTION('center_axis',(0.,1.,0.));
#18539=DIRECTION('ref_axis',(1.,0.,0.));
#18540=DIRECTION('',(0.,1.,0.));
#18541=DIRECTION('center_axis',(0.,1.,0.));
#18542=DIRECTION('ref_axis',(1.,0.,0.));
#18543=DIRECTION('center_axis',(0.,1.,0.));
#18544=DIRECTION('ref_axis',(1.,0.,0.));
#18545=DIRECTION('center_axis',(0.,1.,0.));
#18546=DIRECTION('ref_axis',(1.,0.,0.));
#18547=DIRECTION('center_axis',(0.,1.,0.));
#18548=DIRECTION('ref_axis',(1.,0.,0.));
#18549=DIRECTION('',(0.,1.,0.));
#18550=DIRECTION('center_axis',(0.,1.,0.));
#18551=DIRECTION('ref_axis',(1.,0.,0.));
#18552=DIRECTION('center_axis',(0.,1.,0.));
#18553=DIRECTION('ref_axis',(1.,0.,0.));
#18554=DIRECTION('center_axis',(0.,1.,0.));
#18555=DIRECTION('ref_axis',(1.,0.,0.));
#18556=DIRECTION('',(0.,1.,0.));
#18557=DIRECTION('center_axis',(0.,1.,0.));
#18558=DIRECTION('ref_axis',(1.,0.,0.));
#18559=DIRECTION('',(0.,-1.,0.));
#18560=DIRECTION('center_axis',(0.,-1.,0.));
#18561=DIRECTION('ref_axis',(1.,0.,0.));
#18562=DIRECTION('center_axis',(0.,1.,0.));
#18563=DIRECTION('ref_axis',(1.,0.,0.));
#18564=DIRECTION('',(-1.,0.,0.));
#18565=DIRECTION('center_axis',(0.,1.,0.));
#18566=DIRECTION('ref_axis',(1.,0.,0.));
#18567=DIRECTION('',(-1.,0.,0.));
#18568=DIRECTION('center_axis',(0.,1.,0.));
#18569=DIRECTION('ref_axis',(-1.,0.,0.));
#18570=DIRECTION('',(-1.,0.,0.));
#18571=DIRECTION('',(0.,0.,1.));
#18572=DIRECTION('',(-1.,0.,0.));
#18573=DIRECTION('',(0.,0.,1.));
#18574=DIRECTION('',(-1.,0.,0.));
#18575=DIRECTION('',(0.,0.,1.));
#18576=DIRECTION('',(-1.,0.,0.));
#18577=DIRECTION('',(0.,0.,1.));
#18578=DIRECTION('',(-1.,0.,0.));
#18579=DIRECTION('center_axis',(0.,-1.,0.));
#18580=DIRECTION('ref_axis',(1.,0.,0.));
#18581=DIRECTION('',(-1.,0.,0.));
#18582=DIRECTION('center_axis',(0.,-1.,0.));
#18583=DIRECTION('ref_axis',(1.,0.,0.));
#18584=DIRECTION('',(-1.,0.,0.));
#18585=DIRECTION('center_axis',(0.,-1.,0.));
#18586=DIRECTION('ref_axis',(1.,0.,0.));
#18587=DIRECTION('center_axis',(0.,-1.,0.));
#18588=DIRECTION('ref_axis',(1.,0.,0.));
#18589=DIRECTION('center_axis',(0.,-1.,0.));
#18590=DIRECTION('ref_axis',(1.,0.,0.));
#18591=DIRECTION('center_axis',(0.,-1.,0.));
#18592=DIRECTION('ref_axis',(1.,0.,0.));
#18593=DIRECTION('center_axis',(0.,0.,1.));
#18594=DIRECTION('ref_axis',(1.,0.,0.));
#18595=DIRECTION('',(0.,-1.,0.));
#18596=DIRECTION('',(1.,0.,0.));
#18597=DIRECTION('',(0.,-1.,0.));
#18598=DIRECTION('',(-1.,0.,0.));
#18599=DIRECTION('',(0.,-1.,0.));
#18600=DIRECTION('',(1.,0.,0.));
#18601=DIRECTION('',(0.,-1.,0.));
#18602=DIRECTION('',(1.,0.,0.));
#18603=DIRECTION('',(0.,1.,0.));
#18604=DIRECTION('center_axis',(0.,0.,-1.));
#18605=DIRECTION('ref_axis',(1.,0.,0.));
#18606=DIRECTION('center_axis',(0.,0.,-1.));
#18607=DIRECTION('ref_axis',(1.,0.,0.));
#18608=DIRECTION('center_axis',(0.,0.,-1.));
#18609=DIRECTION('ref_axis',(1.,0.,0.));
#18610=DIRECTION('center_axis',(0.,0.,-1.));
#18611=DIRECTION('ref_axis',(1.,0.,0.));
#18612=DIRECTION('center_axis',(0.,0.,-1.));
#18613=DIRECTION('ref_axis',(1.,0.,0.));
#18614=DIRECTION('center_axis',(0.,1.,0.));
#18615=DIRECTION('ref_axis',(1.,0.,0.));
#18616=DIRECTION('center_axis',(0.,1.,0.));
#18617=DIRECTION('ref_axis',(1.,0.,0.));
#18618=DIRECTION('',(0.,1.,0.));
#18619=DIRECTION('center_axis',(0.,1.,0.));
#18620=DIRECTION('ref_axis',(1.,0.,0.));
#18621=DIRECTION('center_axis',(0.,1.,0.));
#18622=DIRECTION('ref_axis',(1.,0.,0.));
#18623=DIRECTION('center_axis',(0.,-1.,0.));
#18624=DIRECTION('ref_axis',(1.,0.,0.));
#18625=DIRECTION('',(1.,0.,0.));
#18626=DIRECTION('center_axis',(0.,-1.,0.));
#18627=DIRECTION('ref_axis',(1.,0.,0.));
#18628=DIRECTION('',(1.,0.,0.));
#18629=DIRECTION('center_axis',(0.,1.,0.));
#18630=DIRECTION('ref_axis',(1.,0.,0.));
#18631=DIRECTION('',(1.,0.,0.));
#18632=DIRECTION('center_axis',(0.,1.,0.));
#18633=DIRECTION('ref_axis',(1.,0.,0.));
#18634=DIRECTION('',(1.,0.,0.));
#18635=DIRECTION('',(0.,0.,1.));
#18636=DIRECTION('',(1.,0.,0.));
#18637=DIRECTION('',(0.,0.,1.));
#18638=DIRECTION('',(1.,0.,0.));
#18639=DIRECTION('',(0.,0.,1.));
#18640=DIRECTION('',(1.,0.,0.));
#18641=DIRECTION('',(0.,0.,1.));
#18642=DIRECTION('center_axis',(0.,1.,0.));
#18643=DIRECTION('ref_axis',(1.,0.,0.));
#18644=DIRECTION('center_axis',(0.,1.,0.));
#18645=DIRECTION('ref_axis',(1.,0.,0.));
#18646=DIRECTION('center_axis',(0.,1.,0.));
#18647=DIRECTION('ref_axis',(1.,0.,0.));
#18648=DIRECTION('center_axis',(0.,1.,0.));
#18649=DIRECTION('ref_axis',(1.,0.,0.));
#18650=DIRECTION('center_axis',(0.,0.,1.));
#18651=DIRECTION('ref_axis',(1.,0.,0.));
#18652=DIRECTION('',(0.,1.,0.));
#18653=DIRECTION('',(-1.,0.,0.));
#18654=DIRECTION('',(0.,-1.,0.));
#18655=DIRECTION('',(1.,0.,0.));
#18656=DIRECTION('',(0.,-1.,0.));
#18657=DIRECTION('center_axis',(0.,1.,0.));
#18658=DIRECTION('ref_axis',(1.,0.,0.));
#18659=DIRECTION('center_axis',(0.,-1.,0.));
#18660=DIRECTION('ref_axis',(1.,0.,0.));
#18661=DIRECTION('center_axis',(0.,1.,0.));
#18662=DIRECTION('ref_axis',(1.,0.,0.));
#18663=DIRECTION('',(0.,1.,0.));
#18664=DIRECTION('center_axis',(0.,1.,0.));
#18665=DIRECTION('ref_axis',(1.,0.,0.));
#18666=DIRECTION('center_axis',(0.,1.,0.));
#18667=DIRECTION('ref_axis',(-1.,0.,0.));
#18668=DIRECTION('',(1.,0.,0.));
#18669=DIRECTION('center_axis',(0.,1.,0.));
#18670=DIRECTION('ref_axis',(1.,0.,0.));
#18671=DIRECTION('',(1.,0.,0.));
#18672=DIRECTION('center_axis',(0.,1.,0.));
#18673=DIRECTION('ref_axis',(1.,0.,0.));
#18674=DIRECTION('',(1.,0.,0.));
#18675=DIRECTION('',(0.,0.,1.));
#18676=DIRECTION('',(-1.,0.,0.));
#18677=DIRECTION('',(0.,0.,1.));
#18678=DIRECTION('center_axis',(0.,0.,1.));
#18679=DIRECTION('ref_axis',(1.,0.,0.));
#18680=DIRECTION('',(0.,-1.,0.));
#18681=DIRECTION('',(-1.,0.,0.));
#18682=DIRECTION('',(0.,-1.,0.));
#18683=DIRECTION('center_axis',(0.,1.,0.));
#18684=DIRECTION('ref_axis',(1.,0.,0.));
#18685=DIRECTION('center_axis',(0.,1.,0.));
#18686=DIRECTION('ref_axis',(1.,0.,0.));
#18687=DIRECTION('',(0.,1.,0.));
#18688=DIRECTION('center_axis',(0.,1.,0.));
#18689=DIRECTION('ref_axis',(1.,0.,0.));
#18690=DIRECTION('center_axis',(0.,1.,0.));
#18691=DIRECTION('ref_axis',(1.,0.,0.));
#18692=DIRECTION('center_axis',(0.,1.,0.));
#18693=DIRECTION('ref_axis',(1.,0.,0.));
#18694=DIRECTION('',(0.,1.,0.));
#18695=DIRECTION('center_axis',(0.,1.,0.));
#18696=DIRECTION('ref_axis',(1.,0.,0.));
#18697=DIRECTION('center_axis',(0.,1.,0.));
#18698=DIRECTION('ref_axis',(1.,0.,0.));
#18699=DIRECTION('',(0.,1.,0.));
#18700=DIRECTION('center_axis',(0.,1.,0.));
#18701=DIRECTION('ref_axis',(1.,0.,0.));
#18702=DIRECTION('center_axis',(0.,1.,0.));
#18703=DIRECTION('ref_axis',(1.,0.,0.));
#18704=DIRECTION('center_axis',(0.,1.,0.));
#18705=DIRECTION('ref_axis',(1.,0.,0.));
#18706=DIRECTION('',(0.,1.,0.));
#18707=DIRECTION('center_axis',(0.,1.,0.));
#18708=DIRECTION('ref_axis',(1.,0.,0.));
#18709=DIRECTION('center_axis',(0.,1.,0.));
#18710=DIRECTION('ref_axis',(1.,0.,0.));
#18711=DIRECTION('center_axis',(0.,1.,0.));
#18712=DIRECTION('ref_axis',(1.,0.,0.));
#18713=DIRECTION('',(0.,1.,0.));
#18714=DIRECTION('center_axis',(0.,1.,0.));
#18715=DIRECTION('ref_axis',(1.,0.,0.));
#18716=DIRECTION('center_axis',(0.,1.,0.));
#18717=DIRECTION('ref_axis',(1.,0.,0.));
#18718=DIRECTION('',(-1.,0.,0.));
#18719=DIRECTION('center_axis',(0.,1.,0.));
#18720=DIRECTION('ref_axis',(1.,0.,0.));
#18721=DIRECTION('center_axis',(0.,1.,0.));
#18722=DIRECTION('ref_axis',(1.,0.,0.));
#18723=DIRECTION('center_axis',(0.,1.,0.));
#18724=DIRECTION('ref_axis',(1.,0.,0.));
#18725=DIRECTION('',(0.,1.,0.));
#18726=DIRECTION('center_axis',(0.,1.,0.));
#18727=DIRECTION('ref_axis',(1.,0.,0.));
#18728=DIRECTION('center_axis',(0.,-1.,0.));
#18729=DIRECTION('ref_axis',(1.,0.,0.));
#18730=DIRECTION('',(1.,0.,0.));
#18731=DIRECTION('center_axis',(0.,0.,1.));
#18732=DIRECTION('ref_axis',(1.,0.,0.));
#18733=DIRECTION('',(0.,1.,0.));
#18734=DIRECTION('',(-1.,0.,0.));
#18735=DIRECTION('',(0.,-1.,0.));
#18736=DIRECTION('',(1.,0.,0.));
#18737=DIRECTION('',(0.,-1.,0.));
#18738=DIRECTION('center_axis',(0.,1.,0.));
#18739=DIRECTION('ref_axis',(1.,0.,0.));
#18740=DIRECTION('',(0.,1.,0.));
#18741=DIRECTION('center_axis',(0.,1.,0.));
#18742=DIRECTION('ref_axis',(1.,0.,0.));
#18743=DIRECTION('center_axis',(0.,-1.,0.));
#18744=DIRECTION('ref_axis',(1.,0.,0.));
#18745=DIRECTION('center_axis',(0.,-1.,0.));
#18746=DIRECTION('ref_axis',(1.,0.,0.));
#18747=DIRECTION('',(0.,0.,1.));
#18748=DIRECTION('',(1.,0.,0.));
#18749=DIRECTION('',(0.,0.,1.));
#18750=DIRECTION('',(-1.,0.,0.));
#18751=DIRECTION('center_axis',(0.,-1.,0.));
#18752=DIRECTION('ref_axis',(1.,0.,0.));
#18753=DIRECTION('center_axis',(0.,0.,1.));
#18754=DIRECTION('ref_axis',(1.,0.,0.));
#18755=DIRECTION('',(0.,-1.,0.));
#18756=DIRECTION('',(-1.,0.,0.));
#18757=DIRECTION('',(0.,-1.,0.));
#18758=DIRECTION('center_axis',(0.,1.,0.));
#18759=DIRECTION('ref_axis',(1.,0.,0.));
#18760=DIRECTION('center_axis',(0.,1.,0.));
#18761=DIRECTION('ref_axis',(1.,0.,0.));
#18762=DIRECTION('',(0.,1.,0.));
#18763=DIRECTION('center_axis',(0.,1.,0.));
#18764=DIRECTION('ref_axis',(1.,0.,0.));
#18765=DIRECTION('center_axis',(0.,1.,0.));
#18766=DIRECTION('ref_axis',(1.,0.,0.));
#18767=DIRECTION('center_axis',(0.,1.,0.));
#18768=DIRECTION('ref_axis',(1.,0.,0.));
#18769=DIRECTION('',(0.,1.,0.));
#18770=DIRECTION('center_axis',(0.,1.,0.));
#18771=DIRECTION('ref_axis',(1.,0.,0.));
#18772=DIRECTION('center_axis',(0.,1.,0.));
#18773=DIRECTION('ref_axis',(1.,0.,0.));
#18774=DIRECTION('',(0.,1.,0.));
#18775=DIRECTION('center_axis',(0.,1.,0.));
#18776=DIRECTION('ref_axis',(1.,0.,0.));
#18777=DIRECTION('center_axis',(0.,1.,0.));
#18778=DIRECTION('ref_axis',(1.,0.,0.));
#18779=DIRECTION('center_axis',(0.,1.,0.));
#18780=DIRECTION('ref_axis',(1.,0.,0.));
#18781=DIRECTION('',(0.,1.,0.));
#18782=DIRECTION('center_axis',(0.,1.,0.));
#18783=DIRECTION('ref_axis',(1.,0.,0.));
#18784=DIRECTION('center_axis',(0.,1.,0.));
#18785=DIRECTION('ref_axis',(1.,0.,0.));
#18786=DIRECTION('center_axis',(0.,1.,0.));
#18787=DIRECTION('ref_axis',(1.,0.,0.));
#18788=DIRECTION('',(0.,1.,0.));
#18789=DIRECTION('center_axis',(0.,1.,0.));
#18790=DIRECTION('ref_axis',(1.,0.,0.));
#18791=DIRECTION('center_axis',(0.,1.,0.));
#18792=DIRECTION('ref_axis',(1.,0.,0.));
#18793=DIRECTION('',(-1.,0.,0.));
#18794=DIRECTION('center_axis',(0.,1.,0.));
#18795=DIRECTION('ref_axis',(1.,0.,0.));
#18796=DIRECTION('center_axis',(0.,0.,1.));
#18797=DIRECTION('ref_axis',(1.,0.,0.));
#18798=DIRECTION('',(0.,-1.,0.));
#18799=DIRECTION('',(0.,1.,0.));
#18800=DIRECTION('',(1.,0.,0.));
#18801=DIRECTION('',(0.,1.,0.));
#18802=DIRECTION('',(0.,1.,0.));
#18803=DIRECTION('',(0.,1.,0.));
#18804=DIRECTION('center_axis',(0.,0.,-1.));
#18805=DIRECTION('ref_axis',(1.,0.,0.));
#18806=DIRECTION('center_axis',(0.,0.,-1.));
#18807=DIRECTION('ref_axis',(1.,0.,0.));
#18808=DIRECTION('center_axis',(0.,0.,-1.));
#18809=DIRECTION('ref_axis',(1.,0.,0.));
#18810=DIRECTION('center_axis',(0.,0.,-1.));
#18811=DIRECTION('ref_axis',(1.,0.,0.));
#18812=DIRECTION('center_axis',(0.,0.,-1.));
#18813=DIRECTION('ref_axis',(1.,0.,0.));
#18814=DIRECTION('center_axis',(0.,1.,0.));
#18815=DIRECTION('ref_axis',(1.,0.,0.));
#18816=DIRECTION('center_axis',(0.,1.,0.));
#18817=DIRECTION('ref_axis',(1.,0.,0.));
#18818=DIRECTION('center_axis',(0.,1.,0.));
#18819=DIRECTION('ref_axis',(1.,0.,0.));
#18820=DIRECTION('center_axis',(0.,-1.,0.));
#18821=DIRECTION('ref_axis',(1.,0.,0.));
#18822=DIRECTION('center_axis',(0.,1.,0.));
#18823=DIRECTION('ref_axis',(1.,0.,0.));
#18824=DIRECTION('center_axis',(0.,1.,0.));
#18825=DIRECTION('ref_axis',(1.,0.,0.));
#18826=DIRECTION('center_axis',(0.,0.,1.));
#18827=DIRECTION('ref_axis',(1.,0.,0.));
#18828=DIRECTION('center_axis',(0.,0.,1.));
#18829=DIRECTION('ref_axis',(1.,0.,0.));
#18830=DIRECTION('',(0.,0.,1.));
#18831=DIRECTION('center_axis',(0.,0.,-1.));
#18832=DIRECTION('ref_axis',(1.,0.,0.));
#18833=DIRECTION('center_axis',(0.,0.,1.));
#18834=DIRECTION('ref_axis',(1.,0.,0.));
#18835=DIRECTION('center_axis',(0.,0.,1.));
#18836=DIRECTION('ref_axis',(1.,0.,0.));
#18837=DIRECTION('center_axis',(0.,0.,1.));
#18838=DIRECTION('ref_axis',(1.,0.,0.));
#18839=DIRECTION('center_axis',(0.,0.,1.));
#18840=DIRECTION('ref_axis',(1.,0.,0.));
#18841=DIRECTION('',(0.,0.,1.));
#18842=DIRECTION('center_axis',(0.,0.,-1.));
#18843=DIRECTION('ref_axis',(1.,0.,0.));
#18844=DIRECTION('center_axis',(0.,0.,1.));
#18845=DIRECTION('ref_axis',(1.,0.,0.));
#18846=DIRECTION('center_axis',(0.,0.,1.));
#18847=DIRECTION('ref_axis',(1.,0.,0.));
#18848=DIRECTION('center_axis',(0.,0.,1.));
#18849=DIRECTION('ref_axis',(1.,0.,0.));
#18850=DIRECTION('center_axis',(0.,0.,1.));
#18851=DIRECTION('ref_axis',(1.,0.,0.));
#18852=DIRECTION('',(0.,0.,1.));
#18853=DIRECTION('center_axis',(0.,0.,-1.));
#18854=DIRECTION('ref_axis',(1.,0.,0.));
#18855=DIRECTION('center_axis',(0.,0.,1.));
#18856=DIRECTION('ref_axis',(1.,0.,0.));
#18857=DIRECTION('center_axis',(0.,0.,1.));
#18858=DIRECTION('ref_axis',(1.,0.,0.));
#18859=DIRECTION('center_axis',(0.,0.,1.));
#18860=DIRECTION('ref_axis',(1.,0.,0.));
#18861=DIRECTION('center_axis',(0.,0.,1.));
#18862=DIRECTION('ref_axis',(1.,0.,0.));
#18863=DIRECTION('',(0.,0.,1.));
#18864=DIRECTION('center_axis',(0.,0.,-1.));
#18865=DIRECTION('ref_axis',(1.,0.,0.));
#18866=DIRECTION('center_axis',(0.,0.,1.));
#18867=DIRECTION('ref_axis',(1.,0.,0.));
#18868=DIRECTION('center_axis',(0.,0.,1.));
#18869=DIRECTION('ref_axis',(1.,0.,0.));
#18870=DIRECTION('center_axis',(0.,0.,1.));
#18871=DIRECTION('ref_axis',(1.,0.,0.));
#18872=DIRECTION('center_axis',(0.,0.,1.));
#18873=DIRECTION('ref_axis',(1.,0.,0.));
#18874=DIRECTION('',(0.,0.,1.));
#18875=DIRECTION('center_axis',(0.,0.,1.));
#18876=DIRECTION('ref_axis',(1.,0.,0.));
#18877=DIRECTION('center_axis',(0.,0.,1.));
#18878=DIRECTION('ref_axis',(1.,0.,0.));
#18879=DIRECTION('',(0.,0.,1.));
#18880=DIRECTION('center_axis',(0.,0.,1.));
#18881=DIRECTION('ref_axis',(1.,0.,0.));
#18882=DIRECTION('center_axis',(0.,0.,1.));
#18883=DIRECTION('ref_axis',(1.,0.,0.));
#18884=DIRECTION('',(0.,0.,1.));
#18885=DIRECTION('center_axis',(0.,0.,1.));
#18886=DIRECTION('ref_axis',(1.,0.,0.));
#18887=DIRECTION('center_axis',(0.,0.,1.));
#18888=DIRECTION('ref_axis',(1.,0.,0.));
#18889=DIRECTION('',(0.,0.,1.));
#18890=DIRECTION('center_axis',(0.,0.,1.));
#18891=DIRECTION('ref_axis',(1.,0.,0.));
#18892=DIRECTION('center_axis',(0.,0.,1.));
#18893=DIRECTION('ref_axis',(1.,0.,0.));
#18894=DIRECTION('',(0.,0.,1.));
#18895=DIRECTION('center_axis',(0.,0.,1.));
#18896=DIRECTION('ref_axis',(1.,0.,0.));
#18897=DIRECTION('center_axis',(0.,0.,1.));
#18898=DIRECTION('ref_axis',(1.,0.,0.));
#18899=DIRECTION('center_axis',(0.,0.,1.));
#18900=DIRECTION('ref_axis',(1.,0.,0.));
#18901=DIRECTION('',(0.,0.,1.));
#18902=DIRECTION('center_axis',(0.,0.,1.));
#18903=DIRECTION('ref_axis',(1.,0.,0.));
#18904=DIRECTION('center_axis',(0.,0.,1.));
#18905=DIRECTION('ref_axis',(1.,0.,0.));
#18906=DIRECTION('center_axis',(0.,0.,1.));
#18907=DIRECTION('ref_axis',(1.,0.,0.));
#18908=DIRECTION('',(0.,0.,1.));
#18909=DIRECTION('center_axis',(0.,0.,1.));
#18910=DIRECTION('ref_axis',(1.,0.,0.));
#18911=DIRECTION('center_axis',(0.,0.,1.));
#18912=DIRECTION('ref_axis',(1.,0.,0.));
#18913=DIRECTION('center_axis',(0.,0.,1.));
#18914=DIRECTION('ref_axis',(1.,0.,0.));
#18915=DIRECTION('',(0.,0.,1.));
#18916=DIRECTION('center_axis',(0.,0.,1.));
#18917=DIRECTION('ref_axis',(1.,0.,0.));
#18918=DIRECTION('center_axis',(0.,0.,1.));
#18919=DIRECTION('ref_axis',(1.,0.,0.));
#18920=DIRECTION('center_axis',(0.,0.,1.));
#18921=DIRECTION('ref_axis',(1.,0.,0.));
#18922=DIRECTION('',(0.,0.,1.));
#18923=DIRECTION('center_axis',(0.,0.,1.));
#18924=DIRECTION('ref_axis',(1.,0.,0.));
#18925=DIRECTION('center_axis',(0.,0.,1.));
#18926=DIRECTION('ref_axis',(1.,0.,0.));
#18927=DIRECTION('',(0.,0.,1.));
#18928=DIRECTION('center_axis',(0.,0.,1.));
#18929=DIRECTION('ref_axis',(1.,0.,0.));
#18930=DIRECTION('center_axis',(0.,0.,1.));
#18931=DIRECTION('ref_axis',(1.,0.,0.));
#18932=DIRECTION('',(0.,0.,1.));
#18933=DIRECTION('center_axis',(0.,0.,1.));
#18934=DIRECTION('ref_axis',(1.,0.,0.));
#18935=DIRECTION('center_axis',(0.,0.,1.));
#18936=DIRECTION('ref_axis',(1.,0.,0.));
#18937=DIRECTION('',(0.,0.,1.));
#18938=DIRECTION('center_axis',(0.,0.,1.));
#18939=DIRECTION('ref_axis',(1.,0.,0.));
#18940=DIRECTION('center_axis',(0.,0.,1.));
#18941=DIRECTION('ref_axis',(1.,0.,0.));
#18942=DIRECTION('',(0.,0.,1.));
#18943=DIRECTION('center_axis',(0.,0.,1.));
#18944=DIRECTION('ref_axis',(1.,0.,0.));
#18945=DIRECTION('center_axis',(0.,0.,1.));
#18946=DIRECTION('ref_axis',(1.,0.,0.));
#18947=DIRECTION('',(0.,0.,1.));
#18948=DIRECTION('center_axis',(1.,0.,0.));
#18949=DIRECTION('ref_axis',(0.,1.,0.));
#18950=DIRECTION('',(0.,1.,0.));
#18951=DIRECTION('center_axis',(0.,0.,1.));
#18952=DIRECTION('ref_axis',(1.,0.,0.));
#18953=DIRECTION('',(0.,-1.,0.));
#18954=DIRECTION('center_axis',(1.,0.,0.));
#18955=DIRECTION('ref_axis',(0.,1.,0.));
#18956=DIRECTION('',(0.,1.,0.));
#18957=DIRECTION('center_axis',(-1.,0.,0.));
#18958=DIRECTION('ref_axis',(0.,-1.,0.));
#18959=DIRECTION('',(0.,-1.,0.));
#18960=DIRECTION('center_axis',(0.,0.,1.));
#18961=DIRECTION('ref_axis',(1.,0.,0.));
#18962=DIRECTION('',(0.,1.,0.));
#18963=DIRECTION('center_axis',(-1.,0.,0.));
#18964=DIRECTION('ref_axis',(0.,-1.,0.));
#18965=DIRECTION('',(0.,-1.,0.));
#18966=DIRECTION('center_axis',(1.,0.,0.));
#18967=DIRECTION('ref_axis',(0.,1.,0.));
#18968=DIRECTION('',(0.,1.,0.));
#18969=DIRECTION('center_axis',(0.,0.,1.));
#18970=DIRECTION('ref_axis',(1.,0.,0.));
#18971=DIRECTION('center_axis',(-1.,0.,0.));
#18972=DIRECTION('ref_axis',(0.,-1.,0.));
#18973=DIRECTION('',(0.,-1.,0.));
#18974=DIRECTION('center_axis',(0.,0.,1.));
#18975=DIRECTION('ref_axis',(1.,0.,0.));
#22827=CARTESIAN_POINT('',(0.,0.,0.));
#22828=CARTESIAN_POINT('Origin',(10.161522368915,6.1,8.16152236891498));
#22829=CARTESIAN_POINT('',(9.99652236891498,6.1,8.16152236891498));
#22830=CARTESIAN_POINT('Origin',(10.161522368915,6.1,8.16152236891498));
#22831=CARTESIAN_POINT('',(9.99652236891498,7.5,8.16152236891498));
#22832=CARTESIAN_POINT('',(9.99652236891498,6.1,8.16152236891498));
#22833=CARTESIAN_POINT('Origin',(10.161522368915,7.5,8.16152236891498));
#22834=CARTESIAN_POINT('Origin',(10.161522368915,6.1,8.16152236891498));
#22835=CARTESIAN_POINT('Origin',(13.838477631085,6.1,8.16152236891498));
#22836=CARTESIAN_POINT('',(13.673477631085,6.1,8.16152236891498));
#22837=CARTESIAN_POINT('Origin',(13.838477631085,6.1,8.16152236891498));
#22838=CARTESIAN_POINT('',(13.673477631085,7.5,8.16152236891498));
#22839=CARTESIAN_POINT('',(13.673477631085,6.1,8.16152236891498));
#22840=CARTESIAN_POINT('Origin',(13.838477631085,7.5,8.16152236891498));
#22841=CARTESIAN_POINT('Origin',(13.838477631085,6.1,8.16152236891498));
#22842=CARTESIAN_POINT('Origin',(10.161522368915,-7.6,8.16152236891498));
#22843=CARTESIAN_POINT('',(9.99652236891498,-7.5,8.16152236891498));
#22844=CARTESIAN_POINT('Origin',(10.161522368915,-7.5,8.16152236891498));
#22845=CARTESIAN_POINT('',(9.99652236891498,-6.1,8.16152236891498));
#22846=CARTESIAN_POINT('',(9.99652236891498,-7.6,8.16152236891498));
#22847=CARTESIAN_POINT('Origin',(10.161522368915,-6.1,8.16152236891498));
#22848=CARTESIAN_POINT('Origin',(10.161522368915,-6.1,8.16152236891498));
#22849=CARTESIAN_POINT('Origin',(13.838477631085,-7.6,8.16152236891498));
#22850=CARTESIAN_POINT('',(13.673477631085,-7.5,8.16152236891498));
#22851=CARTESIAN_POINT('Origin',(13.838477631085,-7.5,8.16152236891498));
#22852=CARTESIAN_POINT('',(13.673477631085,-6.1,8.16152236891498));
#22853=CARTESIAN_POINT('',(13.673477631085,-7.6,8.16152236891498));
#22854=CARTESIAN_POINT('Origin',(13.838477631085,-6.1,8.16152236891498));
#22855=CARTESIAN_POINT('Origin',(13.838477631085,-6.1,8.16152236891498));
#22856=CARTESIAN_POINT('Origin',(12.,5.3,10.));
#22857=CARTESIAN_POINT('',(9.65,5.3,10.));
#22858=CARTESIAN_POINT('',(9.65,7.5,10.));
#22859=CARTESIAN_POINT('',(9.65,5.3,10.));
#22860=CARTESIAN_POINT('',(14.35,5.3,10.));
#22861=CARTESIAN_POINT('Origin',(12.,5.3,10.));
#22862=CARTESIAN_POINT('',(14.35,7.5,10.));
#22863=CARTESIAN_POINT('',(14.35,5.3,10.));
#22864=CARTESIAN_POINT('Origin',(12.,7.5,10.));
#22865=CARTESIAN_POINT('Origin',(12.,5.3,10.));
#22866=CARTESIAN_POINT('',(10.1,5.3,10.));
#22867=CARTESIAN_POINT('',(9.25,5.3,10.));
#22868=CARTESIAN_POINT('',(13.9,5.3,10.));
#22869=CARTESIAN_POINT('Origin',(12.,5.3,10.));
#22870=CARTESIAN_POINT('',(9.25,5.3,10.));
#22871=CARTESIAN_POINT('Origin',(17.,7.5,1.));
#22872=CARTESIAN_POINT('',(18.5,7.5,10.));
#22873=CARTESIAN_POINT('',(18.5,7.5,10.));
#22874=CARTESIAN_POINT('',(18.5,7.5,9.2));
#22875=CARTESIAN_POINT('',(18.5,7.5,9.2));
#22876=CARTESIAN_POINT('',(17.,7.5,9.2));
#22877=CARTESIAN_POINT('',(18.5,7.5,9.2));
#22878=CARTESIAN_POINT('',(17.,7.5,1.));
#22879=CARTESIAN_POINT('',(17.,7.5,1.));
#22880=CARTESIAN_POINT('',(-4.,7.5,1.));
#22881=CARTESIAN_POINT('',(17.,7.5,1.));
#22882=CARTESIAN_POINT('',(-4.,7.5,9.2));
#22883=CARTESIAN_POINT('',(-4.,7.5,1.));
#22884=CARTESIAN_POINT('',(-5.5,7.5,9.2));
#22885=CARTESIAN_POINT('',(-4.,7.5,9.2));
#22886=CARTESIAN_POINT('',(-5.5,7.5,10.));
#22887=CARTESIAN_POINT('',(-5.5,7.5,9.2));
#22888=CARTESIAN_POINT('',(-1.6,7.5,10.));
#22889=CARTESIAN_POINT('',(18.5,7.5,10.));
#22890=CARTESIAN_POINT('',(1.6,7.5,10.));
#22891=CARTESIAN_POINT('Origin',(0.,7.5,10.));
#22892=CARTESIAN_POINT('',(3.65,7.5,10.));
#22893=CARTESIAN_POINT('',(18.5,7.5,10.));
#22894=CARTESIAN_POINT('',(8.35,7.5,10.));
#22895=CARTESIAN_POINT('Origin',(6.,7.5,10.));
#22896=CARTESIAN_POINT('',(18.5,7.5,10.));
#22897=CARTESIAN_POINT('',(1.24921356237309,7.5,8.5857864376269));
#22898=CARTESIAN_POINT('Origin',(1.41421356237309,7.5,8.5857864376269));
#22899=CARTESIAN_POINT('',(-1.5792135623731,7.5,8.5857864376269));
#22900=CARTESIAN_POINT('Origin',(-1.4142135623731,7.5,8.5857864376269));
#22901=CARTESIAN_POINT('',(7.67347763108502,7.5,8.16152236891498));
#22902=CARTESIAN_POINT('Origin',(7.83847763108502,7.5,8.16152236891498));
#22903=CARTESIAN_POINT('',(3.99652236891498,7.5,8.16152236891498));
#22904=CARTESIAN_POINT('Origin',(4.16152236891498,7.5,8.16152236891498));
#22905=CARTESIAN_POINT('Origin',(6.5,0.,10.));
#22906=CARTESIAN_POINT('',(13.9,5.,10.));
#22907=CARTESIAN_POINT('',(13.9,-7.6,10.));
#22908=CARTESIAN_POINT('',(16.4,5.,10.));
#22909=CARTESIAN_POINT('',(11.45,5.,10.));
#22910=CARTESIAN_POINT('',(16.4,-5.,10.));
#22911=CARTESIAN_POINT('',(16.4,-2.5,10.));
#22912=CARTESIAN_POINT('',(13.9,-5.,10.));
#22913=CARTESIAN_POINT('',(1.65,-5.,10.));
#22914=CARTESIAN_POINT('',(13.9,-5.3,10.));
#22915=CARTESIAN_POINT('',(13.9,-7.6,10.));
#22916=CARTESIAN_POINT('',(14.35,-5.3,10.));
#22917=CARTESIAN_POINT('',(9.25,-5.3,10.));
#22918=CARTESIAN_POINT('',(14.35,-7.5,10.));
#22919=CARTESIAN_POINT('',(14.35,-7.6,10.));
#22920=CARTESIAN_POINT('',(18.5,-7.5,10.));
#22921=CARTESIAN_POINT('',(-5.5,-7.5,10.));
#22922=CARTESIAN_POINT('',(18.5,-7.5,10.));
#22923=CARTESIAN_POINT('',(17.6,3.,10.));
#22924=CARTESIAN_POINT('Origin',(17.75,3.,10.));
#22925=CARTESIAN_POINT('',(17.5,3.06161699786838E-17,10.));
#22926=CARTESIAN_POINT('Origin',(17.75,0.,10.));
#22927=CARTESIAN_POINT('',(17.5,-6.,10.));
#22928=CARTESIAN_POINT('Origin',(17.75,-6.,10.));
#22929=CARTESIAN_POINT('',(17.5,6.,10.));
#22930=CARTESIAN_POINT('Origin',(17.75,6.,10.));
#22931=CARTESIAN_POINT('',(17.6,-3.,10.));
#22932=CARTESIAN_POINT('Origin',(17.75,-3.,10.));
#22933=CARTESIAN_POINT('Origin',(12.,-7.6,10.));
#22934=CARTESIAN_POINT('',(9.65,-5.3,10.));
#22935=CARTESIAN_POINT('Origin',(12.,-5.3,10.));
#22936=CARTESIAN_POINT('',(9.65,-7.5,10.));
#22937=CARTESIAN_POINT('',(9.65,-7.6,10.));
#22938=CARTESIAN_POINT('Origin',(12.,-7.5,10.));
#22939=CARTESIAN_POINT('Origin',(12.,-5.3,10.));
#22940=CARTESIAN_POINT('',(10.1,-5.3,10.));
#22941=CARTESIAN_POINT('Origin',(12.,-5.3,10.));
#22942=CARTESIAN_POINT('',(9.25,-5.3,10.));
#22943=CARTESIAN_POINT('Origin',(-4.,-7.5,1.));
#22944=CARTESIAN_POINT('',(8.35,-7.5,10.));
#22945=CARTESIAN_POINT('',(-5.5,-7.5,10.));
#22946=CARTESIAN_POINT('',(3.65,-7.5,10.));
#22947=CARTESIAN_POINT('Origin',(6.,-7.5,10.));
#22948=CARTESIAN_POINT('',(1.6,-7.5,10.));
#22949=CARTESIAN_POINT('',(-5.5,-7.5,10.));
#22950=CARTESIAN_POINT('',(-1.6,-7.5,10.));
#22951=CARTESIAN_POINT('Origin',(0.,-7.5,10.));
#22952=CARTESIAN_POINT('',(-5.5,-7.5,10.));
#22953=CARTESIAN_POINT('',(-5.5,-7.5,10.));
#22954=CARTESIAN_POINT('',(-5.5,-7.5,9.2));
#22955=CARTESIAN_POINT('',(-5.5,-7.5,9.2));
#22956=CARTESIAN_POINT('',(-4.,-7.5,9.2));
#22957=CARTESIAN_POINT('',(-5.5,-7.5,9.2));
#22958=CARTESIAN_POINT('',(-4.,-7.5,1.));
#22959=CARTESIAN_POINT('',(-4.,-7.5,1.));
#22960=CARTESIAN_POINT('',(17.,-7.5,1.));
#22961=CARTESIAN_POINT('',(-4.,-7.5,1.));
#22962=CARTESIAN_POINT('',(17.,-7.5,9.2));
#22963=CARTESIAN_POINT('',(17.,-7.5,1.));
#22964=CARTESIAN_POINT('',(18.5,-7.5,9.2));
#22965=CARTESIAN_POINT('',(17.,-7.5,9.2));
#22966=CARTESIAN_POINT('',(18.5,-7.5,9.2));
#22967=CARTESIAN_POINT('',(3.99652236891498,-7.5,8.16152236891498));
#22968=CARTESIAN_POINT('Origin',(4.16152236891498,-7.5,8.16152236891498));
#22969=CARTESIAN_POINT('',(7.67347763108502,-7.5,8.16152236891498));
#22970=CARTESIAN_POINT('Origin',(7.83847763108502,-7.5,8.16152236891498));
#22971=CARTESIAN_POINT('',(1.24921356237309,-7.5,8.5857864376269));
#22972=CARTESIAN_POINT('Origin',(1.41421356237309,-7.5,8.5857864376269));
#22973=CARTESIAN_POINT('',(-1.5792135623731,-7.5,8.5857864376269));
#22974=CARTESIAN_POINT('Origin',(-1.4142135623731,-7.5,8.5857864376269));
#22975=CARTESIAN_POINT('Origin',(6.5,0.,10.));
#22976=CARTESIAN_POINT('',(10.1,-5.,10.));
#22977=CARTESIAN_POINT('',(10.1,-7.6,10.));
#22978=CARTESIAN_POINT('',(7.9,-5.,10.));
#22979=CARTESIAN_POINT('',(1.65,-5.,10.));
#22980=CARTESIAN_POINT('',(7.9,-5.3,10.));
#22981=CARTESIAN_POINT('',(7.9,-7.6,10.));
#22982=CARTESIAN_POINT('',(8.35,-5.3,10.));
#22983=CARTESIAN_POINT('',(6.25,-5.3,10.));
#22984=CARTESIAN_POINT('',(8.35,-7.6,10.));
#22985=CARTESIAN_POINT('Origin',(12.,-7.6,10.));
#22986=CARTESIAN_POINT('Origin',(12.,-5.,10.));
#22987=CARTESIAN_POINT('Origin',(12.,-7.6,10.));
#22988=CARTESIAN_POINT('',(10.1,5.,10.));
#22989=CARTESIAN_POINT('',(10.1,-7.6,10.));
#22990=CARTESIAN_POINT('Origin',(12.,5.,10.));
#22991=CARTESIAN_POINT('Origin',(16.4,5.,5.));
#22992=CARTESIAN_POINT('',(7.9,5.,10.));
#22993=CARTESIAN_POINT('',(11.45,5.,10.));
#22994=CARTESIAN_POINT('',(4.1,5.,10.));
#22995=CARTESIAN_POINT('Origin',(6.,5.,10.));
#22996=CARTESIAN_POINT('',(1.2,5.,10.));
#22997=CARTESIAN_POINT('',(11.45,5.,10.));
#22998=CARTESIAN_POINT('',(-1.2,5.,10.));
#22999=CARTESIAN_POINT('Origin',(0.,5.,10.));
#23000=CARTESIAN_POINT('',(-3.2,5.,10.));
#23001=CARTESIAN_POINT('',(11.45,5.,10.));
#23002=CARTESIAN_POINT('',(-3.2,5.,5.));
#23003=CARTESIAN_POINT('',(-3.2,5.,5.));
#23004=CARTESIAN_POINT('',(16.4,5.,5.));
#23005=CARTESIAN_POINT('',(16.4,5.,5.));
#23006=CARTESIAN_POINT('',(16.4,5.,5.));
#23007=CARTESIAN_POINT('Origin',(6.5,0.,10.));
#23008=CARTESIAN_POINT('',(8.35,5.3,10.));
#23009=CARTESIAN_POINT('',(8.35,5.3,10.));
#23010=CARTESIAN_POINT('',(7.9,5.3,10.));
#23011=CARTESIAN_POINT('',(6.25,5.3,10.));
#23012=CARTESIAN_POINT('',(7.9,-7.6,10.));
#23013=CARTESIAN_POINT('Origin',(4.16152236891498,6.1,8.16152236891498));
#23014=CARTESIAN_POINT('',(3.99652236891498,6.1,8.16152236891498));
#23015=CARTESIAN_POINT('Origin',(4.16152236891498,6.1,8.16152236891498));
#23016=CARTESIAN_POINT('',(3.99652236891498,6.1,8.16152236891498));
#23017=CARTESIAN_POINT('Origin',(4.16152236891498,6.1,8.16152236891498));
#23018=CARTESIAN_POINT('Origin',(7.83847763108502,6.1,8.16152236891498));
#23019=CARTESIAN_POINT('',(7.67347763108502,6.1,8.16152236891498));
#23020=CARTESIAN_POINT('Origin',(7.83847763108502,6.1,8.16152236891498));
#23021=CARTESIAN_POINT('',(7.67347763108502,6.1,8.16152236891498));
#23022=CARTESIAN_POINT('Origin',(7.83847763108502,6.1,8.16152236891498));
#23023=CARTESIAN_POINT('Origin',(4.16152236891498,-7.6,8.16152236891498));
#23024=CARTESIAN_POINT('',(3.99652236891498,-6.1,8.16152236891498));
#23025=CARTESIAN_POINT('',(3.99652236891498,-7.6,8.16152236891498));
#23026=CARTESIAN_POINT('Origin',(4.16152236891498,-6.1,8.16152236891498));
#23027=CARTESIAN_POINT('Origin',(4.16152236891498,-6.1,8.16152236891498));
#23028=CARTESIAN_POINT('Origin',(7.83847763108502,-7.6,8.16152236891498));
#23029=CARTESIAN_POINT('',(7.67347763108502,-6.1,8.16152236891498));
#23030=CARTESIAN_POINT('',(7.67347763108502,-7.6,8.16152236891498));
#23031=CARTESIAN_POINT('Origin',(7.83847763108502,-6.1,8.16152236891498));
#23032=CARTESIAN_POINT('Origin',(7.83847763108502,-6.1,8.16152236891498));
#23033=CARTESIAN_POINT('Origin',(6.,5.3,10.));
#23034=CARTESIAN_POINT('',(3.65,5.3,10.));
#23035=CARTESIAN_POINT('',(3.65,5.3,10.));
#23036=CARTESIAN_POINT('Origin',(6.,5.3,10.));
#23037=CARTESIAN_POINT('Origin',(6.,5.3,10.));
#23038=CARTESIAN_POINT('',(4.1,5.3,10.));
#23039=CARTESIAN_POINT('',(6.25,5.3,10.));
#23040=CARTESIAN_POINT('Origin',(6.,5.3,10.));
#23041=CARTESIAN_POINT('Origin',(6.,-7.6,10.));
#23042=CARTESIAN_POINT('',(3.65,-5.3,10.));
#23043=CARTESIAN_POINT('Origin',(6.,-5.3,10.));
#23044=CARTESIAN_POINT('',(3.65,-7.6,10.));
#23045=CARTESIAN_POINT('Origin',(6.,-5.3,10.));
#23046=CARTESIAN_POINT('',(4.1,-5.3,10.));
#23047=CARTESIAN_POINT('Origin',(6.,-5.3,10.));
#23048=CARTESIAN_POINT('',(6.25,-5.3,10.));
#23049=CARTESIAN_POINT('Origin',(6.5,0.,10.));
#23050=CARTESIAN_POINT('',(4.1,-5.,10.));
#23051=CARTESIAN_POINT('',(4.1,-7.6,10.));
#23052=CARTESIAN_POINT('',(1.2,-5.,10.));
#23053=CARTESIAN_POINT('',(1.65,-5.,10.));
#23054=CARTESIAN_POINT('',(1.2,-5.5,10.));
#23055=CARTESIAN_POINT('',(1.2,-7.6,10.));
#23056=CARTESIAN_POINT('',(1.6,-5.5,10.));
#23057=CARTESIAN_POINT('',(3.25,-5.5,10.));
#23058=CARTESIAN_POINT('',(1.6,-7.6,10.));
#23059=CARTESIAN_POINT('Origin',(6.,-7.6,10.));
#23060=CARTESIAN_POINT('',(4.1,-7.6,10.));
#23061=CARTESIAN_POINT('Origin',(6.,-7.6,10.));
#23062=CARTESIAN_POINT('Origin',(6.,-5.,10.));
#23063=CARTESIAN_POINT('Origin',(-3.2,-5.,5.));
#23064=CARTESIAN_POINT('',(16.4,-5.,5.));
#23065=CARTESIAN_POINT('',(16.4,-5.,5.));
#23066=CARTESIAN_POINT('',(-3.2,-5.,5.));
#23067=CARTESIAN_POINT('',(-3.2,-5.,5.));
#23068=CARTESIAN_POINT('',(-3.2,-5.,10.));
#23069=CARTESIAN_POINT('',(-3.2,-5.,5.));
#23070=CARTESIAN_POINT('',(-1.2,-5.,10.));
#23071=CARTESIAN_POINT('',(1.65,-5.,10.));
#23072=CARTESIAN_POINT('Origin',(0.,-5.,10.));
#23073=CARTESIAN_POINT('Origin',(6.5,0.,10.));
#23074=CARTESIAN_POINT('',(1.6,5.5,10.));
#23075=CARTESIAN_POINT('',(1.6,5.5,10.));
#23076=CARTESIAN_POINT('',(1.2,5.5,10.));
#23077=CARTESIAN_POINT('',(3.25,5.5,10.));
#23078=CARTESIAN_POINT('',(1.2,-7.6,10.));
#23079=CARTESIAN_POINT('Origin',(-1.4142135623731,6.1,8.5857864376269));
#23080=CARTESIAN_POINT('',(-1.5792135623731,6.1,8.5857864376269));
#23081=CARTESIAN_POINT('Origin',(-1.4142135623731,6.1,8.5857864376269));
#23082=CARTESIAN_POINT('',(-1.5792135623731,6.1,8.5857864376269));
#23083=CARTESIAN_POINT('Origin',(-1.4142135623731,6.1,8.5857864376269));
#23084=CARTESIAN_POINT('Origin',(1.41421356237309,6.1,8.5857864376269));
#23085=CARTESIAN_POINT('',(1.24921356237309,6.1,8.5857864376269));
#23086=CARTESIAN_POINT('Origin',(1.41421356237309,6.1,8.5857864376269));
#23087=CARTESIAN_POINT('',(1.24921356237309,6.1,8.5857864376269));
#23088=CARTESIAN_POINT('Origin',(1.41421356237309,6.1,8.5857864376269));
#23089=CARTESIAN_POINT('Origin',(-1.4142135623731,-7.6,8.5857864376269));
#23090=CARTESIAN_POINT('',(-1.5792135623731,-6.1,8.5857864376269));
#23091=CARTESIAN_POINT('',(-1.5792135623731,-7.6,8.5857864376269));
#23092=CARTESIAN_POINT('Origin',(-1.4142135623731,-6.1,8.5857864376269));
#23093=CARTESIAN_POINT('Origin',(-1.4142135623731,-6.1,8.5857864376269));
#23094=CARTESIAN_POINT('Origin',(1.41421356237309,-7.6,8.5857864376269));
#23095=CARTESIAN_POINT('',(1.24921356237309,-6.1,8.5857864376269));
#23096=CARTESIAN_POINT('',(1.24921356237309,-7.6,8.5857864376269));
#23097=CARTESIAN_POINT('Origin',(1.41421356237309,-6.1,8.5857864376269));
#23098=CARTESIAN_POINT('Origin',(1.41421356237309,-6.1,8.5857864376269));
#23099=CARTESIAN_POINT('Origin',(0.,5.5,10.));
#23100=CARTESIAN_POINT('',(-1.6,5.5,10.));
#23101=CARTESIAN_POINT('',(-1.6,5.5,10.));
#23102=CARTESIAN_POINT('Origin',(0.,5.5,10.));
#23103=CARTESIAN_POINT('Origin',(0.,5.5,10.));
#23104=CARTESIAN_POINT('',(-1.2,5.5,10.));
#23105=CARTESIAN_POINT('',(3.25,5.5,10.));
#23106=CARTESIAN_POINT('Origin',(0.,5.5,10.));
#23107=CARTESIAN_POINT('Origin',(6.5,0.,10.));
#23108=CARTESIAN_POINT('',(-5.5,7.5,10.));
#23109=CARTESIAN_POINT('',(-1.6,-5.5,10.));
#23110=CARTESIAN_POINT('',(-1.6,-7.6,10.));
#23111=CARTESIAN_POINT('',(-1.2,-5.5,10.));
#23112=CARTESIAN_POINT('',(3.25,-5.5,10.));
#23113=CARTESIAN_POINT('',(-1.2,-7.6,10.));
#23114=CARTESIAN_POINT('',(-3.2,2.5,10.));
#23115=CARTESIAN_POINT('',(-1.2,-7.6,10.));
#23116=CARTESIAN_POINT('',(-4.9,3.,10.));
#23117=CARTESIAN_POINT('Origin',(-4.75,3.,10.));
#23118=CARTESIAN_POINT('',(-5.,-6.,10.));
#23119=CARTESIAN_POINT('Origin',(-4.75,-6.,10.));
#23120=CARTESIAN_POINT('',(-5.,3.06161699786838E-17,10.));
#23121=CARTESIAN_POINT('Origin',(-4.75,0.,10.));
#23122=CARTESIAN_POINT('',(-5.,6.,10.));
#23123=CARTESIAN_POINT('Origin',(-4.75,6.,10.));
#23124=CARTESIAN_POINT('',(-4.9,-3.,10.));
#23125=CARTESIAN_POINT('Origin',(-4.75,-3.,10.));
#23126=CARTESIAN_POINT('Origin',(0.,-7.6,10.));
#23127=CARTESIAN_POINT('Origin',(0.,-5.5,10.));
#23128=CARTESIAN_POINT('Origin',(0.,-5.5,10.));
#23129=CARTESIAN_POINT('Origin',(0.,-5.5,10.));
#23130=CARTESIAN_POINT('Origin',(0.,-7.6,10.));
#23131=CARTESIAN_POINT('Origin',(0.,-7.6,10.));
#23132=CARTESIAN_POINT('Origin',(15.,-3.5,1.8));
#23133=CARTESIAN_POINT('',(14.4,-3.5,1.8));
#23134=CARTESIAN_POINT('Origin',(15.,-3.5,1.8));
#23135=CARTESIAN_POINT('',(14.4,-3.5,5.));
#23136=CARTESIAN_POINT('',(14.4,-3.5,1.8));
#23137=CARTESIAN_POINT('Origin',(15.,-3.5,5.));
#23138=CARTESIAN_POINT('Origin',(15.,-3.5,1.8));
#23139=CARTESIAN_POINT('',(14.67,-3.5,1.8));
#23140=CARTESIAN_POINT('Origin',(15.,-3.5,1.8));
#23141=CARTESIAN_POINT('Origin',(-2.,3.5,1.8));
#23142=CARTESIAN_POINT('',(-2.6,3.5,1.8));
#23143=CARTESIAN_POINT('Origin',(-2.,3.5,1.8));
#23144=CARTESIAN_POINT('',(-2.6,3.5,5.));
#23145=CARTESIAN_POINT('',(-2.6,3.5,1.8));
#23146=CARTESIAN_POINT('Origin',(-2.,3.5,5.));
#23147=CARTESIAN_POINT('Origin',(-2.,3.5,1.8));
#23148=CARTESIAN_POINT('',(-2.33,3.5,1.8));
#23149=CARTESIAN_POINT('Origin',(-2.,3.5,1.8));
#23150=CARTESIAN_POINT('Origin',(-2.,-3.5,1.8));
#23151=CARTESIAN_POINT('',(-2.6,-3.5,1.8));
#23152=CARTESIAN_POINT('Origin',(-2.,-3.5,1.8));
#23153=CARTESIAN_POINT('',(-2.6,-3.5,5.));
#23154=CARTESIAN_POINT('',(-2.6,-3.5,1.8));
#23155=CARTESIAN_POINT('Origin',(-2.,-3.5,5.));
#23156=CARTESIAN_POINT('Origin',(-2.,-3.5,1.8));
#23157=CARTESIAN_POINT('',(-2.33,-3.5,1.8));
#23158=CARTESIAN_POINT('Origin',(-2.,-3.5,1.8));
#23159=CARTESIAN_POINT('Origin',(15.,3.5,1.8));
#23160=CARTESIAN_POINT('',(14.4,3.5,1.8));
#23161=CARTESIAN_POINT('Origin',(15.,3.5,1.8));
#23162=CARTESIAN_POINT('',(14.4,3.5,5.));
#23163=CARTESIAN_POINT('',(14.4,3.5,1.8));
#23164=CARTESIAN_POINT('Origin',(15.,3.5,5.));
#23165=CARTESIAN_POINT('Origin',(15.,3.5,1.8));
#23166=CARTESIAN_POINT('',(14.67,3.5,1.8));
#23167=CARTESIAN_POINT('Origin',(15.,3.5,1.8));
#23168=CARTESIAN_POINT('Origin',(15.,-3.5,0.9));
#23169=CARTESIAN_POINT('',(14.67,-3.5,1.));
#23170=CARTESIAN_POINT('Origin',(15.,-3.5,1.));
#23171=CARTESIAN_POINT('',(14.67,-3.5,0.9));
#23172=CARTESIAN_POINT('Origin',(-2.,3.5,0.9));
#23173=CARTESIAN_POINT('',(-2.33,3.5,1.));
#23174=CARTESIAN_POINT('Origin',(-2.,3.5,1.));
#23175=CARTESIAN_POINT('',(-2.33,3.5,0.9));
#23176=CARTESIAN_POINT('Origin',(-2.,-3.5,0.9));
#23177=CARTESIAN_POINT('',(-2.33,-3.5,1.));
#23178=CARTESIAN_POINT('Origin',(-2.,-3.5,1.));
#23179=CARTESIAN_POINT('',(-2.33,-3.5,0.9));
#23180=CARTESIAN_POINT('Origin',(15.,3.5,0.9));
#23181=CARTESIAN_POINT('',(14.67,3.5,1.));
#23182=CARTESIAN_POINT('Origin',(15.,3.5,1.));
#23183=CARTESIAN_POINT('',(14.67,3.5,0.9));
#23184=CARTESIAN_POINT('Origin',(17.75,3.,9.5));
#23185=CARTESIAN_POINT('',(17.6,3.,9.5));
#23186=CARTESIAN_POINT('Origin',(17.75,3.,9.5));
#23187=CARTESIAN_POINT('',(17.6,3.,9.5));
#23188=CARTESIAN_POINT('Origin',(17.75,3.,9.5));
#23189=CARTESIAN_POINT('Origin',(17.75,-3.,9.5));
#23190=CARTESIAN_POINT('',(17.6,-3.,9.5));
#23191=CARTESIAN_POINT('Origin',(17.75,-3.,9.5));
#23192=CARTESIAN_POINT('',(17.6,-3.,9.5));
#23193=CARTESIAN_POINT('Origin',(17.75,-3.,9.5));
#23194=CARTESIAN_POINT('Origin',(-4.75,3.,9.5));
#23195=CARTESIAN_POINT('',(-4.9,3.,9.5));
#23196=CARTESIAN_POINT('Origin',(-4.75,3.,9.5));
#23197=CARTESIAN_POINT('',(-4.9,3.,9.5));
#23198=CARTESIAN_POINT('Origin',(-4.75,3.,9.5));
#23199=CARTESIAN_POINT('Origin',(-4.75,-3.,9.5));
#23200=CARTESIAN_POINT('',(-4.9,-3.,9.5));
#23201=CARTESIAN_POINT('Origin',(-4.75,-3.,9.5));
#23202=CARTESIAN_POINT('',(-4.9,-3.,9.5));
#23203=CARTESIAN_POINT('Origin',(-4.75,-3.,9.5));
#23204=CARTESIAN_POINT('Origin',(17.75,0.,9.1));
#23205=CARTESIAN_POINT('',(17.5,-3.06161699786838E-17,9.2));
#23206=CARTESIAN_POINT('Origin',(17.75,0.,9.2));
#23207=CARTESIAN_POINT('',(17.5,-3.06161699786838E-17,9.1));
#23208=CARTESIAN_POINT('Origin',(-4.75,-6.,9.1));
#23209=CARTESIAN_POINT('',(-5.,-6.,9.2));
#23210=CARTESIAN_POINT('Origin',(-4.75,-6.,9.2));
#23211=CARTESIAN_POINT('',(-5.,-6.,9.1));
#23212=CARTESIAN_POINT('Origin',(-4.75,0.,9.1));
#23213=CARTESIAN_POINT('',(-5.,-3.06161699786838E-17,9.2));
#23214=CARTESIAN_POINT('Origin',(-4.75,0.,9.2));
#23215=CARTESIAN_POINT('',(-5.,-3.06161699786838E-17,9.1));
#23216=CARTESIAN_POINT('Origin',(-4.75,6.,9.1));
#23217=CARTESIAN_POINT('',(-5.,6.,9.2));
#23218=CARTESIAN_POINT('Origin',(-4.75,6.,9.2));
#23219=CARTESIAN_POINT('',(-5.,6.,9.1));
#23220=CARTESIAN_POINT('Origin',(17.75,-6.,9.1));
#23221=CARTESIAN_POINT('',(17.5,-6.,9.2));
#23222=CARTESIAN_POINT('Origin',(17.75,-6.,9.2));
#23223=CARTESIAN_POINT('',(17.5,-6.,9.1));
#23224=CARTESIAN_POINT('Origin',(17.75,6.,9.1));
#23225=CARTESIAN_POINT('',(17.5,6.,9.2));
#23226=CARTESIAN_POINT('Origin',(17.75,6.,9.2));
#23227=CARTESIAN_POINT('',(17.5,6.,9.1));
#23228=CARTESIAN_POINT('Origin',(18.5,-7.5,9.2));
#23229=CARTESIAN_POINT('',(18.5,-7.5,9.2));
#23230=CARTESIAN_POINT('Origin',(17.75,0.,9.2));
#23231=CARTESIAN_POINT('',(17.,-3.75,9.2));
#23232=CARTESIAN_POINT('Origin',(17.,-7.5,1.));
#23233=CARTESIAN_POINT('',(17.,-7.5,1.));
#23234=CARTESIAN_POINT('Origin',(-5.5,7.5,9.2));
#23235=CARTESIAN_POINT('',(-5.5,7.5,9.2));
#23236=CARTESIAN_POINT('Origin',(-4.75,0.,9.2));
#23237=CARTESIAN_POINT('',(-4.,3.75,9.2));
#23238=CARTESIAN_POINT('Origin',(-3.2,5.,5.));
#23239=CARTESIAN_POINT('',(-3.2,5.,5.));
#23240=CARTESIAN_POINT('Origin',(16.4,-5.,5.));
#23241=CARTESIAN_POINT('',(16.4,-5.,5.));
#23242=CARTESIAN_POINT('Origin',(6.6,0.,5.));
#23243=CARTESIAN_POINT('Origin',(-4.,7.5,1.));
#23244=CARTESIAN_POINT('',(-4.,7.5,1.));
#23245=CARTESIAN_POINT('Origin',(6.5,0.,1.));
#73242=UNCERTAINTY_MEASURE_WITH_UNIT(LENGTH_MEASURE(0.001),#73367,
'DISTANCE_ACCURACY_VALUE',
'Maximum model space distance between geometric entities at asserted c
onnectivities');
#73302=UNCERTAINTY_MEASURE_WITH_UNIT(LENGTH_MEASURE(0.001),#73367,
'DISTANCE_ACCURACY_VALUE',
'Maximum model space distance between geometric entities at asserted c
onnectivities');
#73306=(
GEOMETRIC_REPRESENTATION_CONTEXT(3)
GLOBAL_UNCERTAINTY_ASSIGNED_CONTEXT((#73242))
GLOBAL_UNIT_ASSIGNED_CONTEXT((#73367,#73369,#73370))
REPRESENTATION_CONTEXT('','3D')
);
#73366=(
GEOMETRIC_REPRESENTATION_CONTEXT(3)
GLOBAL_UNCERTAINTY_ASSIGNED_CONTEXT((#73302))
GLOBAL_UNIT_ASSIGNED_CONTEXT((#73367,#73369,#73370))
REPRESENTATION_CONTEXT('','3D')
);
#73367=(
LENGTH_UNIT()
NAMED_UNIT(*)
SI_UNIT(.CENTI.,.METRE.)
);
#73369=(
NAMED_UNIT(*)
PLANE_ANGLE_UNIT()
SI_UNIT($,.RADIAN.)
);
#73370=(
NAMED_UNIT(*)
SI_UNIT($,.STERADIAN.)
SOLID_ANGLE_UNIT()
);
#73374=SHAPE_DEFINITION_REPRESENTATION(#73437,#73610);
#73437=PRODUCT_DEFINITION_SHAPE('',$,#73674);
#73610=SHAPE_REPRESENTATION('',(#16833),#73306);
#73670=PRODUCT_DEFINITION_CONTEXT('part definition',#73861,'design');
#73674=PRODUCT_DEFINITION('Lower housing','Lower housing',#73737,#73670);
#73737=PRODUCT_DEFINITION_FORMATION('',$,#73866);
#73861=APPLICATION_CONTEXT(
'Core Data for Automotive Mechanical Design Process');
#73862=PRODUCT_CONTEXT('part definition',#73861,'mechanical');
#73866=PRODUCT('Lower housing','Lower housing','Lower housing',(#73862));
#73961=COLOUR_RGB('Dark Blue',0.08,0.2,0.34);
#73962=FILL_AREA_STYLE_COLOUR('',#73961);
#73963=FILL_AREA_STYLE('',(#73962));
#73964=SURFACE_STYLE_FILL_AREA(#73963);
#73965=SURFACE_SIDE_STYLE('',(#73964));
#73966=SURFACE_STYLE_USAGE(.BOTH.,#73965);
#73967=PRESENTATION_STYLE_ASSIGNMENT((#73966));
ENDSEC;
END-ISO-10303-21;
